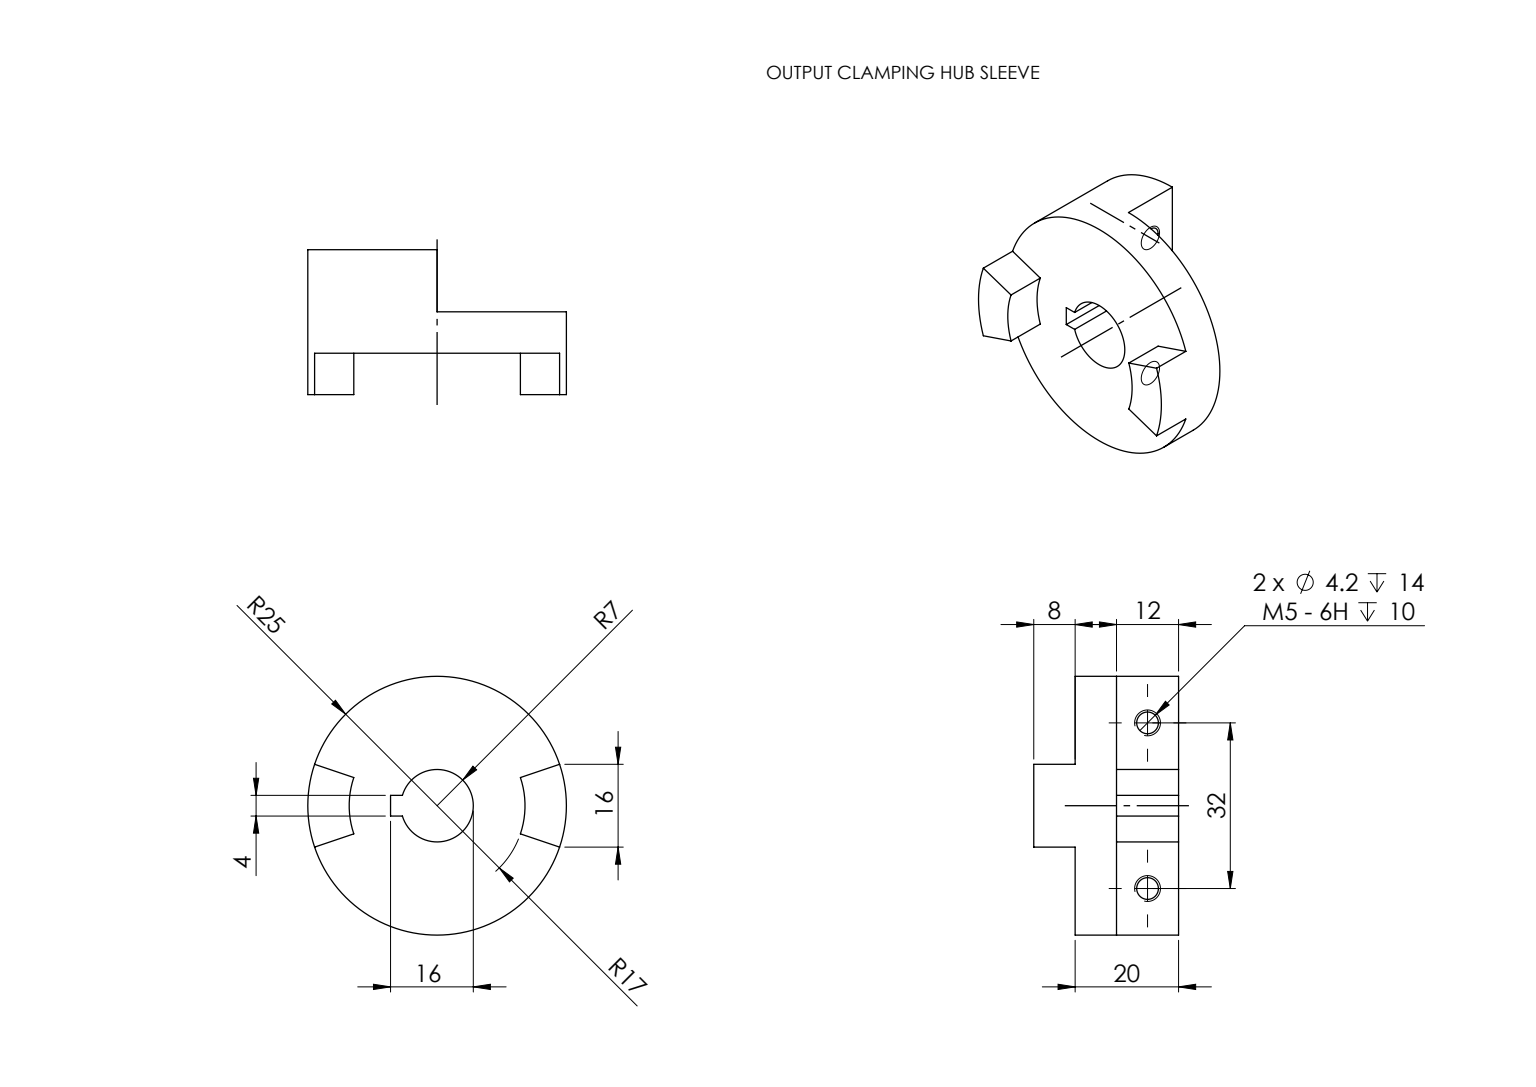
ISO-10303-21;
HEADER;
FILE_DESCRIPTION (('STEP AP214'),
    '1' );
FILE_NAME ('Output Clamping Hub Sleeve.step',
    '2026-10-08T14:09:18',
    ( '' ),
    ( '' ),
    'SwSTEP 2.0',
    'SolidWorks 2026',
    '' );
FILE_SCHEMA (( 'AUTOMOTIVE_DESIGN' ));
ENDSEC;

DATA;
#2=CARTESIAN_POINT ( 'NONE',  ( -6.517431832507181422E-14, 16.00000000000000000, -26.00000000000000355 ) ) ;
#4=CARTESIAN_POINT ( 'NONE',  ( 0.000000000000000000, 0.000000000000000000, -12.00000000000000000 ) ) ;
#5=AXIS2_PLACEMENT_3D ( 'NONE', #3716, #3077, #4925 ) ;
#9=VERTEX_POINT ( 'NONE', #2215 ) ;
#26=FACE_OUTER_BOUND ( 'NONE', #3587, .T. ) ;
#42=ORIENTED_EDGE ( 'NONE', *, *, #4705, .F. ) ;
#48=EDGE_LOOP ( 'NONE', ( #130, #2080, #1685, #2442 ) ) ;
#49=LINE ( 'NONE', #3799, #2903 ) ;
#54=VERTEX_POINT ( 'NONE', #3686 ) ;
#58=FACE_OUTER_BOUND ( 'NONE', #389, .T. ) ;
#82=ORIENTED_EDGE ( 'NONE', *, *, #1120, .T. ) ;
#83=AXIS2_PLACEMENT_3D ( 'NONE', #3595, #2177, #3698 ) ;
#84=ORIENTED_EDGE ( 'NONE', *, *, #4675, .T. ) ;
#85=SURFACE_STYLE_FILL_AREA ( #4292 ) ;
#95=ORIENTED_EDGE ( 'NONE', *, *, #1051, .F. ) ;
#97=VECTOR ( 'NONE', #3015, 1000.000000000000000 ) ;
#100=CIRCLE ( 'NONE', #2908, 6.999999999999999112 ) ;
#103=VECTOR ( 'NONE', #177, 1000.000000000000114 ) ;
#109=CIRCLE ( 'NONE', #436, 17.00000000000000000 ) ;
#112=CARTESIAN_POINT ( 'NONE',  ( 0.000000000000000000, 0.000000000000000000, -20.00000000000000000 ) ) ;
#116=CARTESIAN_POINT ( 'NONE',  ( -25.00000000000000000, 3.061616997868383043E-15, -4.000000000000000000 ) ) ;
#121=VERTEX_POINT ( 'NONE', #126 ) ;
#124=CARTESIAN_POINT ( 'NONE',  ( 16.10609822396473945, -5.439999999999995062, -4.000000000000000000 ) ) ;
#126=CARTESIAN_POINT ( 'NONE',  ( -16.10609822396473945, -5.439999999999995062, -12.00000000000000000 ) ) ;
#130=ORIENTED_EDGE ( 'NONE', *, *, #800, .F. ) ;
#135=DIRECTION ( 'NONE',  ( 0.5150380749100544886, 0.000000000000000000, -0.8571673007021121116 ) ) ;
#143=ORIENTED_EDGE ( 'NONE', *, *, #299, .T. ) ;
#144=DIRECTION ( 'NONE',  ( 1.000000000000000000, -0.000000000000000000, -0.000000000000000000 ) ) ;
#148=VERTEX_POINT ( 'NONE', #905 ) ;
#150=DIRECTION ( 'NONE',  ( -1.000000000000000000, -4.073394895316987600E-15, 0.000000000000000000 ) ) ;
#151=LINE ( 'NONE', #2483, #3855 ) ;
#161=DIRECTION ( 'NONE',  ( -1.000000000000000000, 0.000000000000000000, -0.000000000000000000 ) ) ;
#168=CARTESIAN_POINT ( 'NONE',  ( 23.68543856465402442, -8.000000000000003553, 14.30577747056276472 ) ) ;
#170=ORIENTED_EDGE ( 'NONE', *, *, #708, .F. ) ;
#171=CIRCLE ( 'NONE', #2417, 17.00000000000000000 ) ;
#174=EDGE_CURVE ( 'NONE', #4395, #54, #1471, .T. ) ;
#175=DIRECTION ( 'NONE',  ( 0.9474175425861609545, -0.3199999999999996181, 0.000000000000000000 ) ) ;
#177=DIRECTION ( 'NONE',  ( -0.9474175425861605104, 0.3200000000000010059, 0.000000000000000000 ) ) ;
#185=CARTESIAN_POINT ( 'NONE',  ( 16.10609822396473945, -5.439999999999995062, 14.30577747056276472 ) ) ;
#187=AXIS2_PLACEMENT_3D ( 'NONE', #4125, #819, #1824 ) ;
#189=ORIENTED_EDGE ( 'NONE', *, *, #3151, .T. ) ;
#194=DIRECTION ( 'NONE',  ( 0.000000000000000000, 0.000000000000000000, -1.000000000000000000 ) ) ;
#195=DIRECTION ( 'NONE',  ( -0.9474175425861605104, 0.3200000000000010059, 0.000000000000000000 ) ) ;
#196=EDGE_CURVE ( 'NONE', #2273, #1203, #931, .T. ) ;
#202=MECHANICAL_DESIGN_GEOMETRIC_PRESENTATION_REPRESENTATION('',(#2202),#282);
#210=DIRECTION ( 'NONE',  ( 0.000000000000000000, 0.000000000000000000, -1.000000000000000000 ) ) ;
#217=CARTESIAN_POINT ( 'NONE',  ( -13.99999999999993250, -16.00000000000000000, -26.00000000000000355 ) ) ;
#226=ORIENTED_EDGE ( 'NONE', *, *, #3828, .F. ) ;
#236=VECTOR ( 'NONE', #1592, 1000.000000000000000 ) ;
#238=DIRECTION ( 'NONE',  ( 1.000000000000000000, -0.000000000000000000, -0.000000000000000000 ) ) ;
#242=AXIS2_PLACEMENT_3D ( 'NONE', #3899, #3088, #3132 ) ;
#245=CIRCLE ( 'NONE', #405, 25.00000000000000000 ) ;
#251=DIRECTION ( 'NONE',  ( 1.000000000000000000, 0.000000000000000000, -0.000000000000000000 ) ) ;
#253=CIRCLE ( 'NONE', #5, 2.099999999999997868 ) ;
#254=AXIS2_PLACEMENT_3D ( 'NONE', #4822, #3198, #2921 ) ;
#261=AXIS2_PLACEMENT_3D ( 'NONE', #1866, #4851, #4564 ) ;
#265=( NAMED_UNIT ( * ) PLANE_ANGLE_UNIT ( ) SI_UNIT ( $, .RADIAN. ) );
#267=DIRECTION ( 'NONE',  ( 0.000000000000000000, -1.000000000000000000, 0.000000000000000000 ) ) ;
#269=LINE ( 'NONE', #4370, #3848 ) ;
#277=CARTESIAN_POINT ( 'NONE',  ( 0.000000000000000000, 0.000000000000000000, -12.00000000000000000 ) ) ;
#279=AXIS2_PLACEMENT_3D ( 'NONE', #4796, #2900, #4321 ) ;
#282=( GEOMETRIC_REPRESENTATION_CONTEXT ( 3 ) GLOBAL_UNCERTAINTY_ASSIGNED_CONTEXT ( ( #2248 ) ) GLOBAL_UNIT_ASSIGNED_CONTEXT ( ( #695, #1844, #4603 ) ) REPRESENTATION_CONTEXT ( 'NONE', 'WORKASPACE' ) );
#286=ORIENTED_EDGE ( 'NONE', *, *, #2509, .T. ) ;
#288=EDGE_CURVE ( 'NONE', #1390, #3410, #3646, .T. ) ;
#299=EDGE_CURVE ( 'NONE', #4175, #811, #2955, .T. ) ;
#319=PLANE ( 'NONE',  #4799 ) ;
#323=EDGE_CURVE ( 'NONE', #1722, #1339, #2532, .T. ) ;
#324=EDGE_LOOP ( 'NONE', ( #3270, #945 ) ) ;
#326=CARTESIAN_POINT ( 'NONE',  ( 0.000000000000000000, 25.00000000000000000, -20.00000000000000000 ) ) ;
#336=CARTESIAN_POINT ( 'NONE',  ( -7.332110811570578784E-14, -6.999999999999999112, -32.00000000000000000 ) ) ;
#344=FACE_OUTER_BOUND ( 'NONE', #964, .T. ) ;
#351=DIRECTION ( 'NONE',  ( 0.9474175425861605104, 0.3200000000000010059, 0.000000000000000000 ) ) ;
#353=SURFACE_STYLE_FILL_AREA ( #4217 ) ;
#357=DIRECTION ( 'NONE',  ( 0.9474175425861609545, 0.3199999999999996181, -0.000000000000000000 ) ) ;
#359=DIRECTION ( 'NONE',  ( -0.000000000000000000, -0.000000000000000000, 1.000000000000000000 ) ) ;
#367=ORIENTED_EDGE ( 'NONE', *, *, #4173, .F. ) ;
#378=DIRECTION ( 'NONE',  ( 1.000000000000000000, -0.000000000000000000, -0.000000000000000000 ) ) ;
#388=ORIENTED_EDGE ( 'NONE', *, *, #3153, .T. ) ;
#389=EDGE_LOOP ( 'NONE', ( #2947, #665, #449, #3173, #4854, #2496, #2657, #940, #4548 ) ) ;
#396=CIRCLE ( 'NONE', #2236, 25.00000000000000000 ) ;
#399=CIRCLE ( 'NONE', #3208, 2.099999999999997868 ) ;
#405=AXIS2_PLACEMENT_3D ( 'NONE', #4519, #1873, #1469 ) ;
#407=VECTOR ( 'NONE', #816, 1000.000000000000000 ) ;
#411=CARTESIAN_POINT ( 'NONE',  ( 0.000000000000000000, 0.000000000000000000, -20.00000000000000000 ) ) ;
#413=AXIS2_PLACEMENT_3D ( 'NONE', #411, #1607, #4207 ) ;
#415=ORIENTED_EDGE ( 'NONE', *, *, #196, .T. ) ;
#419=DIRECTION ( 'NONE',  ( -0.000000000000000000, -0.000000000000000000, -1.000000000000000000 ) ) ;
#425=MANIFOLD_SOLID_BREP ( 'M5 Tapped Hole1', #4581 ) ;
#431=DIRECTION ( 'NONE',  ( 0.000000000000000000, 0.000000000000000000, -1.000000000000000000 ) ) ;
#436=AXIS2_PLACEMENT_3D ( 'NONE', #2401, #1271, #4371 ) ;
#449=ORIENTED_EDGE ( 'NONE', *, *, #2315, .T. ) ;
#460=ORIENTED_EDGE ( 'NONE', *, *, #523, .T. ) ;
#462=EDGE_CURVE ( 'NONE', #3903, #3640, #245, .T. ) ;
#469=ADVANCED_BREP_SHAPE_REPRESENTATION ( '', ( #425, #1918 ), #4450 ) ;
#474=( NAMED_UNIT ( * ) SI_UNIT ( $, .STERADIAN. ) SOLID_ANGLE_UNIT ( ) );
#476=DIRECTION ( 'NONE',  ( 0.000000000000000000, 0.000000000000000000, -1.000000000000000000 ) ) ;
#479=VERTEX_POINT ( 'NONE', #1438 ) ;
#483=ADVANCED_FACE ( 'NONE', ( #2985 ), #1043, .F. ) ;
#491=ORIENTED_EDGE ( 'NONE', *, *, #4912, .F. ) ;
#495=LINE ( 'NONE', #1938, #2572 ) ;
#496=CYLINDRICAL_SURFACE ( 'NONE', #2581, 6.999999999999999112 ) ;
#498=AXIS2_PLACEMENT_3D ( 'NONE', #873, #431, #3187 ) ;
#502=DIRECTION ( 'NONE',  ( -0.000000000000000000, -0.000000000000000000, 1.000000000000000000 ) ) ;
#507=DIRECTION ( 'NONE',  ( -1.000000000000000000, 0.000000000000000000, 0.000000000000000000 ) ) ;
#509=ORIENTED_EDGE ( 'NONE', *, *, #4882, .F. ) ;
#511=CIRCLE ( 'NONE', #1053, 6.999999999999999112 ) ;
#518=CIRCLE ( 'NONE', #1149, 17.00000000000000000 ) ;
#520=DIRECTION ( 'NONE',  ( 0.000000000000000000, 0.000000000000000000, -1.000000000000000000 ) ) ;
#523=EDGE_CURVE ( 'NONE', #852, #654, #2199, .T. ) ;
#524=ORIENTED_EDGE ( 'NONE', *, *, #2305, .F. ) ;
#530=ORIENTED_EDGE ( 'NONE', *, *, #1162, .F. ) ;
#536=VERTEX_POINT ( 'NONE', #1955 ) ;
#537=VERTEX_POINT ( 'NONE', #3576 ) ;
#544=( NAMED_UNIT ( * ) PLANE_ANGLE_UNIT ( ) SI_UNIT ( $, .RADIAN. ) );
#545=PLANE ( 'NONE',  #2901 ) ;
#546=DIRECTION ( 'NONE',  ( -0.000000000000000000, -0.000000000000000000, 1.000000000000000000 ) ) ;
#551=CARTESIAN_POINT ( 'NONE',  ( -7.332110811570578784E-14, -6.999999999999999112, -32.00000000000000000 ) ) ;
#554=DIRECTION ( 'NONE',  ( -0.9474175425861605104, -0.3200000000000010059, 0.000000000000000000 ) ) ;
#561=DIRECTION ( 'NONE',  ( 1.000000000000000000, -1.892318758829013864E-15, 0.000000000000000000 ) ) ;
#565=CARTESIAN_POINT ( 'NONE',  ( 23.68543856465402442, -8.000000000000003553, -4.000000000000000000 ) ) ;
#567=ORIENTED_EDGE ( 'NONE', *, *, #4261, .F. ) ;
#573=CARTESIAN_POINT ( 'NONE',  ( -17.00000000000000000, 0.000000000000000000, 14.30577747056276472 ) ) ;
#576=VECTOR ( 'NONE', #357, 1000.000000000000114 ) ;
#579=AXIS2_PLACEMENT_3D ( 'NONE', #2046, #3223, #4745 ) ;
#584=EDGE_LOOP ( 'NONE', ( #3424, #607, #226, #4068, #1963 ) ) ;
#589=ORIENTED_EDGE ( 'NONE', *, *, #3682, .F. ) ;
#593=CARTESIAN_POINT ( 'NONE',  ( -9.000000000000001776, 2.000000000000000000, -20.00000000000000000 ) ) ;
#597=VERTEX_POINT ( 'NONE', #124 ) ;
#600=PRODUCT_CONTEXT ( 'NONE', #768, 'mechanical' ) ;
#607=ORIENTED_EDGE ( 'NONE', *, *, #1884, .F. ) ;
#611=DIRECTION ( 'NONE',  ( -1.000000000000000000, 0.000000000000000000, 0.000000000000000000 ) ) ;
#624=LINE ( 'NONE', #3677, #576 ) ;
#626=LINE ( 'NONE', #4130, #2829 ) ;
#627=ORIENTED_EDGE ( 'NONE', *, *, #2610, .F. ) ;
#630=( LENGTH_UNIT ( ) NAMED_UNIT ( * ) SI_UNIT ( .MILLI., .METRE. ) );
#631=CIRCLE ( 'NONE', #3433, 25.00000000000000000 ) ;
#633=CARTESIAN_POINT ( 'NONE',  ( -6.517431832507181422E-14, 16.00000000000000000, -28.10000000000000142 ) ) ;
#637=DIRECTION ( 'NONE',  ( 0.000000000000000000, 0.000000000000000000, -1.000000000000000000 ) ) ;
#642=CARTESIAN_POINT ( 'NONE',  ( -13.99999999999993250, -16.00000000000000000, -26.00000000000000355 ) ) ;
#653=CIRCLE ( 'NONE', #3857, 2.099999999999997868 ) ;
#654=VERTEX_POINT ( 'NONE', #4651 ) ;
#658=PLANE ( 'NONE',  #2178 ) ;
#659=AXIS2_PLACEMENT_3D ( 'NONE', #1459, #3001, #4158 ) ;
#665=ORIENTED_EDGE ( 'NONE', *, *, #2003, .T. ) ;
#674=COLOUR_RGB ( '', 0.09019608, 0.27058824, 0.51372549) ;
#689=CARTESIAN_POINT ( 'NONE',  ( 16.10609822396473589, 5.440000000000003055, -4.000000000000000000 ) ) ;
#694=DIRECTION ( 'NONE',  ( 0.000000000000000000, 0.000000000000000000, -1.000000000000000000 ) ) ;
#695=( LENGTH_UNIT ( ) NAMED_UNIT ( * ) SI_UNIT ( .MILLI., .METRE. ) );
#701=ORIENTED_EDGE ( 'NONE', *, *, #4533, .T. ) ;
#707=ORIENTED_EDGE ( 'NONE', *, *, #765, .F. ) ;
#708=EDGE_CURVE ( 'NONE', #2396, #2782, #2504, .T. ) ;
#713=AXIS2_PLACEMENT_3D ( 'NONE', #1995, #4324, #507 ) ;
#720=VECTOR ( 'NONE', #1698, 1000.000000000000000 ) ;
#724=CARTESIAN_POINT ( 'NONE',  ( 6.497531322021036645E-14, -16.00000000000000000, -23.90000000000000568 ) ) ;
#731=DIRECTION ( 'NONE',  ( -0.000000000000000000, -0.000000000000000000, 1.000000000000000000 ) ) ;
#757=CARTESIAN_POINT ( 'NONE',  ( 0.000000000000000000, -1.999999999999999112, -20.00000000000000000 ) ) ;
#758=CYLINDRICAL_SURFACE ( 'NONE', #3930, 2.099999999999997868 ) ;
#765=EDGE_CURVE ( 'NONE', #148, #1558, #1764, .T. ) ;
#768=APPLICATION_CONTEXT ( 'automotive_design' ) ;
#782=ORIENTED_EDGE ( 'NONE', *, *, #2643, .T. ) ;
#790=UNCERTAINTY_MEASURE_WITH_UNIT (LENGTH_MEASURE( 1.000000000000000082E-05 ), #921, 'distance_accuracy_value', 'NONE');
#800=EDGE_CURVE ( 'NONE', #3536, #4716, #4237, .T. ) ;
#806=DIRECTION ( 'NONE',  ( -0.000000000000000000, -0.000000000000000000, 1.000000000000000000 ) ) ;
#809=VECTOR ( 'NONE', #2774, 1000.000000000000000 ) ;
#811=VERTEX_POINT ( 'NONE', #4516 ) ;
#815=CIRCLE ( 'NONE', #1850, 2.099999999999997868 ) ;
#816=DIRECTION ( 'NONE',  ( 0.5150380749100544886, 1.049727191138618449E-16, 0.8571673007021121116 ) ) ;
#819=DIRECTION ( 'NONE',  ( 0.000000000000000000, 0.000000000000000000, 1.000000000000000000 ) ) ;
#822=VECTOR ( 'NONE', #3608, 1000.000000000000114 ) ;
#850=LINE ( 'NONE', #4216, #4959 ) ;
#852=VERTEX_POINT ( 'NONE', #2573 ) ;
#865=VERTEX_POINT ( 'NONE', #3009 ) ;
#867=DIRECTION ( 'NONE',  ( 1.000000000000000000, -0.000000000000000000, -0.000000000000000000 ) ) ;
#873=CARTESIAN_POINT ( 'NONE',  ( 0.000000000000000000, 0.000000000000000000, -20.00000000000000000 ) ) ;
#891=CARTESIAN_POINT ( 'NONE',  ( 0.000000000000000000, 0.000000000000000000, -12.00000000000000000 ) ) ;
#897=DIRECTION ( 'NONE',  ( -0.000000000000000000, -0.000000000000000000, -1.000000000000000000 ) ) ;
#901=VECTOR ( 'NONE', #135, 1000.000000000000000 ) ;
#903=ORIENTED_EDGE ( 'NONE', *, *, #1204, .T. ) ;
#905=CARTESIAN_POINT ( 'NONE',  ( 23.68543856465402442, -8.000000000000003553, -4.000000000000000000 ) ) ;
#910=LINE ( 'NONE', #1678, #1139 ) ;
#911=EDGE_LOOP ( 'NONE', ( #4750, #2184, #415, #388 ) ) ;
#921=( LENGTH_UNIT ( ) NAMED_UNIT ( * ) SI_UNIT ( .MILLI., .METRE. ) );
#927=CARTESIAN_POINT ( 'NONE',  ( -9.000000000000003553, -1.999999999999999112, -12.00000000000000000 ) ) ;
#931=LINE ( 'NONE', #2457, #3169 ) ;
#937=LINE ( 'NONE', #3914, #2427 ) ;
#940=ORIENTED_EDGE ( 'NONE', *, *, #4943, .T. ) ;
#945=ORIENTED_EDGE ( 'NONE', *, *, #2751, .F. ) ;
#948=ORIENTED_EDGE ( 'NONE', *, *, #4220, .T. ) ;
#951=CARTESIAN_POINT ( 'NONE',  ( -6.537332342993324937E-14, 16.00000000000000000, -26.00000000000000355 ) ) ;
#962=DIRECTION ( 'NONE',  ( 0.000000000000000000, 0.000000000000000000, -1.000000000000000000 ) ) ;
#964=EDGE_LOOP ( 'NONE', ( #3898, #1479, #2019, #627, #4843, #4193 ) ) ;
#968=CIRCLE ( 'NONE', #4077, 25.00000000000000000 ) ;
#969=ORIENTED_EDGE ( 'NONE', *, *, #1204, .F. ) ;
#974=CARTESIAN_POINT ( 'NONE',  ( 0.000000000000000000, 0.000000000000000000, -12.00000000000000000 ) ) ;
#977=ORIENTED_EDGE ( 'NONE', *, *, #4608, .F. ) ;
#984=LINE ( 'NONE', #4405, #3775 ) ;
#991=VERTEX_POINT ( 'NONE', #116 ) ;
#1000=CARTESIAN_POINT ( 'NONE',  ( 16.10609822396473589, 5.440000000000003055, 14.30577747056276472 ) ) ;
#1007=CARTESIAN_POINT ( 'NONE',  ( -6.537332342993324937E-14, 16.00000000000000000, -26.00000000000000355 ) ) ;
#1016=PRODUCT ( 'Output Clamping Hub Sleeve', 'Output Clamping Hub Sleeve', '', ( #600 ) ) ;
#1017=CYLINDRICAL_SURFACE ( 'NONE', #1512, 17.00000000000000000 ) ;
#1021=MECHANICAL_DESIGN_GEOMETRIC_PRESENTATION_REPRESENTATION('',(#3423),#4138);
#1027=EDGE_CURVE ( 'NONE', #3993, #1343, #968, .T. ) ;
#1029=PLANE ( 'NONE',  #4821 ) ;
#1031=VERTEX_POINT ( 'NONE', #4319 ) ;
#1035=DIRECTION ( 'NONE',  ( 1.000000000000000000, -0.000000000000000000, -0.000000000000000000 ) ) ;
#1038=EDGE_LOOP ( 'NONE', ( #524, #589, #4148, #2680, #1210, #4780, #1790, #3348, #2804, #82 ) ) ;
#1041=DIRECTION ( 'NONE',  ( -0.000000000000000000, -0.000000000000000000, 1.000000000000000000 ) ) ;
#1043=CONICAL_SURFACE ( 'NONE', #1362, 2.099999999999997868, 1.029744258676654090 ) ;
#1051=EDGE_CURVE ( 'NONE', #1467, #479, #3496, .T. ) ;
#1053=AXIS2_PLACEMENT_3D ( 'NONE', #974, #3260, #3214 ) ;
#1058=AXIS2_PLACEMENT_3D ( 'NONE', #3400, #2679, #251 ) ;
#1063=CARTESIAN_POINT ( 'NONE',  ( -16.10609822396473589, 5.440000000000003055, -4.000000000000000000 ) ) ;
#1079=CARTESIAN_POINT ( 'NONE',  ( 0.000000000000000000, 25.00000000000000000, -32.00000000000000000 ) ) ;
#1082=FACE_OUTER_BOUND ( 'NONE', #3709, .T. ) ;
#1083=EDGE_LOOP ( 'NONE', ( #286, #4197, #170, #2268 ) ) ;
#1087=FACE_OUTER_BOUND ( 'NONE', #1306, .T. ) ;
#1090=ORIENTED_EDGE ( 'NONE', *, *, #3059, .T. ) ;
#1115=DIRECTION ( 'NONE',  ( 1.000000000000000000, 0.000000000000000000, 0.000000000000000000 ) ) ;
#1118=AXIS2_PLACEMENT_3D ( 'NONE', #3796, #3850, #2357 ) ;
#1120=EDGE_CURVE ( 'NONE', #1203, #991, #1604, .T. ) ;
#1122=DIRECTION ( 'NONE',  ( -0.000000000000000000, -0.000000000000000000, 1.000000000000000000 ) ) ;
#1139=VECTOR ( 'NONE', #2847, 1000.000000000000000 ) ;
#1144=AXIS2_PLACEMENT_3D ( 'NONE', #891, #2352, #3950 ) ;
#1146=CARTESIAN_POINT ( 'NONE',  ( 0.000000000000000000, 0.000000000000000000, 0.000000000000000000 ) ) ;
#1148=FACE_OUTER_BOUND ( 'NONE', #3721, .T. ) ;
#1149=AXIS2_PLACEMENT_3D ( 'NONE', #2228, #1470, #1993 ) ;
#1151=CYLINDRICAL_SURFACE ( 'NONE', #3829, 25.00000000000000000 ) ;
#1152=FILL_AREA_STYLE_COLOUR ( '', #674 ) ;
#1162=EDGE_CURVE ( 'NONE', #4131, #3536, #1946, .T. ) ;
#1170=EDGE_LOOP ( 'NONE', ( #1550, #3395, #4871, #3982 ) ) ;
#1171=CARTESIAN_POINT ( 'NONE',  ( 0.000000000000000000, 0.000000000000000000, -4.000000000000000000 ) ) ;
#1173=PLANE ( 'NONE',  #187 ) ;
#1178=ADVANCED_FACE ( 'NONE', ( #2145 ), #4808, .F. ) ;
#1182=EDGE_CURVE ( 'NONE', #4937, #2834, #3660, .T. ) ;
#1188=COLOUR_RGB ( '', 0.09019608, 0.27058824, 0.51372549) ;
#1203=VERTEX_POINT ( 'NONE', #4060 ) ;
#1204=EDGE_CURVE ( 'NONE', #1722, #1390, #2521, .T. ) ;
#1210=ORIENTED_EDGE ( 'NONE', *, *, #4882, .T. ) ;
#1215=DIRECTION ( 'NONE',  ( -0.000000000000000000, -0.000000000000000000, 1.000000000000000000 ) ) ;
#1223=FACE_OUTER_BOUND ( 'NONE', #4578, .T. ) ;
#1227=AXIS2_PLACEMENT_3D ( 'NONE', #2025, #867, #476 ) ;
#1228=FACE_OUTER_BOUND ( 'NONE', #3061, .T. ) ;
#1244=LINE ( 'NONE', #2091, #822 ) ;
#1261=ORIENTED_EDGE ( 'NONE', *, *, #3181, .T. ) ;
#1264=DIRECTION ( 'NONE',  ( 4.073394895316987600E-15, -1.000000000000000000, 0.000000000000000000 ) ) ;
#1266=EDGE_LOOP ( 'NONE', ( #3202, #3863, #2347, #3636 ) ) ;
#1271=DIRECTION ( 'NONE',  ( 0.000000000000000000, 0.000000000000000000, 1.000000000000000000 ) ) ;
#1284=AXIS2_PLACEMENT_3D ( 'NONE', #4119, #4902, #2527 ) ;
#1285=ORIENTED_EDGE ( 'NONE', *, *, #4911, .F. ) ;
#1289=FACE_OUTER_BOUND ( 'NONE', #4132, .T. ) ;
#1292=ORIENTED_EDGE ( 'NONE', *, *, #2610, .T. ) ;
#1293=CARTESIAN_POINT ( 'NONE',  ( -14.00000000000006395, 16.00000000000000000, -26.00000000000000355 ) ) ;
#1298=ORIENTED_EDGE ( 'NONE', *, *, #2437, .T. ) ;
#1305=CIRCLE ( 'NONE', #1144, 25.00000000000000000 ) ;
#1306=EDGE_LOOP ( 'NONE', ( #4774, #1285, #3515, #1292 ) ) ;
#1316=EDGE_CURVE ( 'NONE', #2020, #1912, #4082, .T. ) ;
#1319=VERTEX_POINT ( 'NONE', #3970 ) ;
#1329=ADVANCED_FACE ( 'NONE', ( #2541 ), #545, .T. ) ;
#1336=FACE_OUTER_BOUND ( 'NONE', #4607, .T. ) ;
#1339=VERTEX_POINT ( 'NONE', #1063 ) ;
#1341=CARTESIAN_POINT ( 'NONE',  ( -13.99999999999993250, -16.00000000000000000, -26.00000000000000355 ) ) ;
#1343=VERTEX_POINT ( 'NONE', #4509 ) ;
#1355=ORIENTED_EDGE ( 'NONE', *, *, #3411, .T. ) ;
#1362=AXIS2_PLACEMENT_3D ( 'NONE', #1897, #3377, #2606 ) ;
#1364=CARTESIAN_POINT ( 'NONE',  ( 25.00000000000000000, 0.000000000000000000, -20.00000000000000000 ) ) ;
#1368=CIRCLE ( 'NONE', #2824, 6.999999999999999112 ) ;
#1376=AXIS2_PLACEMENT_3D ( 'NONE', #3753, #4202, #3409 ) ;
#1377=APPLICATION_CONTEXT ( 'automotive_design' ) ;
#1387=DIRECTION ( 'NONE',  ( 0.000000000000000000, 0.000000000000000000, -1.000000000000000000 ) ) ;
#1389=DIRECTION ( 'NONE',  ( 1.000000000000000000, -0.000000000000000000, -0.000000000000000000 ) ) ;
#1390=VERTEX_POINT ( 'NONE', #2638 ) ;
#1412=CYLINDRICAL_SURFACE ( 'NONE', #261, 6.999999999999999112 ) ;
#1421=ADVANCED_FACE ( 'NONE', ( #3392 ), #658, .F. ) ;
#1433=FACE_OUTER_BOUND ( 'NONE', #1585, .T. ) ;
#1436=ORIENTED_EDGE ( 'NONE', *, *, #1447, .F. ) ;
#1438=CARTESIAN_POINT ( 'NONE',  ( 6.497531322021036645E-14, -16.00000000000000000, -28.10000000000000142 ) ) ;
#1441=VECTOR ( 'NONE', #3616, 1000.000000000000000 ) ;
#1447=EDGE_CURVE ( 'NONE', #2396, #654, #4893, .T. ) ;
#1451=CARTESIAN_POINT ( 'NONE',  ( 2.444036937190193033E-14, 6.999999999999999112, -20.00000000000000000 ) ) ;
#1455=EDGE_LOOP ( 'NONE', ( #42, #2415, #3096, #2460 ) ) ;
#1457=AXIS2_PLACEMENT_3D ( 'NONE', #1971, #2989, #3498 ) ;
#1459=CARTESIAN_POINT ( 'NONE',  ( -4.336808689942023652E-16, 2.000000000000002220, -20.00000000000000000 ) ) ;
#1467=VERTEX_POINT ( 'NONE', #3787 ) ;
#1469=DIRECTION ( 'NONE',  ( -1.000000000000000000, 0.000000000000000000, 0.000000000000000000 ) ) ;
#1470=DIRECTION ( 'NONE',  ( 0.000000000000000000, 0.000000000000000000, 1.000000000000000000 ) ) ;
#1471=CIRCLE ( 'NONE', #4031, 6.999999999999999112 ) ;
#1473=LINE ( 'NONE', #326, #97 ) ;
#1479=ORIENTED_EDGE ( 'NONE', *, *, #4639, .T. ) ;
#1499=ORIENTED_EDGE ( 'NONE', *, *, #299, .F. ) ;
#1512=AXIS2_PLACEMENT_3D ( 'NONE', #2201, #637, #3326 ) ;
#1522=DIRECTION ( 'NONE',  ( -1.000000000000000000, -3.784637517658031179E-16, -0.000000000000000000 ) ) ;
#1531=DIRECTION ( 'NONE',  ( 0.000000000000000000, 0.000000000000000000, -1.000000000000000000 ) ) ;
#1550=ORIENTED_EDGE ( 'NONE', *, *, #4235, .T. ) ;
#1555=PLANE ( 'NONE',  #2113 ) ;
#1557=LINE ( 'NONE', #4611, #4253 ) ;
#1558=VERTEX_POINT ( 'NONE', #4592 ) ;
#1562=DIRECTION ( 'NONE',  ( -1.000000000000000000, 0.000000000000000000, -0.000000000000000000 ) ) ;
#1567=ORIENTED_EDGE ( 'NONE', *, *, #1945, .F. ) ;
#1578=DIRECTION ( 'NONE',  ( 1.000000000000000000, 2.168404344971009361E-16, 0.000000000000000000 ) ) ;
#1583=CARTESIAN_POINT ( 'NONE',  ( -7.332110811570578784E-14, -6.999999999999999112, -20.00000000000000000 ) ) ;
#1585=EDGE_LOOP ( 'NONE', ( #1499, #1942, #2195, #3333 ) ) ;
#1592=DIRECTION ( 'NONE',  ( 1.000000000000000000, -0.000000000000000000, -0.000000000000000000 ) ) ;
#1599=CARTESIAN_POINT ( 'NONE',  ( -4.336808689942023652E-16, 2.000000000000002220, -12.00000000000000000 ) ) ;
#1604=CIRCLE ( 'NONE', #3762, 25.00000000000000000 ) ;
#1607=DIRECTION ( 'NONE',  ( -0.000000000000000000, -0.000000000000000000, 1.000000000000000000 ) ) ;
#1614=SURFACE_SIDE_STYLE ('',( #85 ) ) ;
#1630=DIRECTION ( 'NONE',  ( 4.073394895316987600E-15, -1.000000000000000000, 0.000000000000000000 ) ) ;
#1645=EDGE_CURVE ( 'NONE', #1339, #3410, #2044, .T. ) ;
#1647=DIRECTION ( 'NONE',  ( -0.000000000000000000, -0.000000000000000000, -1.000000000000000000 ) ) ;
#1653=LINE ( 'NONE', #4734, #103 ) ;
#1660=ORIENTED_EDGE ( 'NONE', *, *, #1996, .T. ) ;
#1669=EDGE_CURVE ( 'NONE', #597, #1031, #1681, .T. ) ;
#1672=EDGE_LOOP ( 'NONE', ( #3004, #3131, #3882, #3418 ) ) ;
#1678=CARTESIAN_POINT ( 'NONE',  ( -23.68543856465402442, -8.000000000000003553, 14.30577747056276472 ) ) ;
#1681=LINE ( 'NONE', #185, #1934 ) ;
#1685=ORIENTED_EDGE ( 'NONE', *, *, #2751, .T. ) ;
#1690=DIRECTION ( 'NONE',  ( -1.000000000000000000, 0.000000000000000000, 0.000000000000000000 ) ) ;
#1691=VECTOR ( 'NONE', #731, 1000.000000000000000 ) ;
#1697=DIRECTION ( 'NONE',  ( 1.357798298438996130E-15, -1.000000000000000000, 0.000000000000000000 ) ) ;
#1698=DIRECTION ( 'NONE',  ( 4.073394895316987600E-15, -1.000000000000000000, 0.000000000000000000 ) ) ;
#1715=VECTOR ( 'NONE', #2134, 1000.000000000000114 ) ;
#1722=VERTEX_POINT ( 'NONE', #4383 ) ;
#1729=DIRECTION ( 'NONE',  ( -4.336808689942018722E-16, -1.000000000000000000, 0.000000000000000000 ) ) ;
#1735=FACE_OUTER_BOUND ( 'NONE', #1170, .T. ) ;
#1757=FACE_OUTER_BOUND ( 'NONE', #3032, .T. ) ;
#1760=EDGE_LOOP ( 'NONE', ( #189, #4344, #367, #1298 ) ) ;
#1764=LINE ( 'NONE', #168, #1840 ) ;
#1774=PRODUCT_DEFINITION_SHAPE ( 'NONE', 'NONE',  #2896 ) ;
#1775=ORIENTED_EDGE ( 'NONE', *, *, #323, .T. ) ;
#1781=DIRECTION ( 'NONE',  ( 1.000000000000000000, -0.000000000000000000, -0.000000000000000000 ) ) ;
#1783=CIRCLE ( 'NONE', #2761, 25.00000000000000000 ) ;
#1786=CARTESIAN_POINT ( 'NONE',  ( 0.000000000000000000, 0.000000000000000000, -12.00000000000000000 ) ) ;
#1790=ORIENTED_EDGE ( 'NONE', *, *, #765, .T. ) ;
#1794=DIRECTION ( 'NONE',  ( 1.000000000000000000, -0.000000000000000000, -0.000000000000000000 ) ) ;
#1803=LINE ( 'NONE', #3332, #2185 ) ;
#1810=( NAMED_UNIT ( * ) SI_UNIT ( $, .STERADIAN. ) SOLID_ANGLE_UNIT ( ) );
#1814=CARTESIAN_POINT ( 'NONE',  ( 2.444036937190193033E-14, 6.999999999999999112, -32.00000000000000000 ) ) ;
#1824=DIRECTION ( 'NONE',  ( 1.000000000000000000, 0.000000000000000000, -0.000000000000000000 ) ) ;
#1836=DIRECTION ( 'NONE',  ( 0.000000000000000000, 0.000000000000000000, -1.000000000000000000 ) ) ;
#1840=VECTOR ( 'NONE', #4831, 1000.000000000000000 ) ;
#1844=( NAMED_UNIT ( * ) PLANE_ANGLE_UNIT ( ) SI_UNIT ( $, .RADIAN. ) );
#1850=AXIS2_PLACEMENT_3D ( 'NONE', #1007, #3965, #2141 ) ;
#1852=PLANE ( 'NONE',  #2825 ) ;
#1853=ADVANCED_FACE ( 'NONE', ( #4885, #2557 ), #1852, .F. ) ;
#1857=VECTOR ( 'NONE', #1522, 1000.000000000000000 ) ;
#1866=CARTESIAN_POINT ( 'NONE',  ( 0.000000000000000000, 0.000000000000000000, -20.00000000000000000 ) ) ;
#1872=CARTESIAN_POINT ( 'NONE',  ( -6.708203932499367639, 2.000000000000001332, -32.00000000000000000 ) ) ;
#1873=DIRECTION ( 'NONE',  ( 0.000000000000000000, 0.000000000000000000, -1.000000000000000000 ) ) ;
#1879=DIRECTION ( 'NONE',  ( -1.000000000000000000, 0.000000000000000000, 0.000000000000000000 ) ) ;
#1884=EDGE_CURVE ( 'NONE', #4842, #3993, #624, .T. ) ;
#1897=CARTESIAN_POINT ( 'NONE',  ( -13.99999999999993250, -16.00000000000000000, -26.00000000000000355 ) ) ;
#1909=CARTESIAN_POINT ( 'NONE',  ( 0.000000000000000000, 0.000000000000000000, -12.00000000000000000 ) ) ;
#1910=EDGE_CURVE ( 'NONE', #3903, #4259, #1473, .T. ) ;
#1912=VERTEX_POINT ( 'NONE', #4524 ) ;
#1914=ORIENTED_EDGE ( 'NONE', *, *, #4729, .T. ) ;
#1918=AXIS2_PLACEMENT_3D ( 'NONE', #1146, #2700, #1115 ) ;
#1920=DIRECTION ( 'NONE',  ( -0.000000000000000000, -0.000000000000000000, 1.000000000000000000 ) ) ;
#1929=CARTESIAN_POINT ( 'NONE',  ( -16.10609822396473589, 5.440000000000003055, -12.00000000000000000 ) ) ;
#1934=VECTOR ( 'NONE', #520, 1000.000000000000000 ) ;
#1938=CARTESIAN_POINT ( 'NONE',  ( -1.387778780781444295E-15, 4.108768631691174362E-15, -12.00000000000000000 ) ) ;
#1942=ORIENTED_EDGE ( 'NONE', *, *, #3742, .T. ) ;
#1945=EDGE_CURVE ( 'NONE', #3993, #4372, #49, .T. ) ;
#1946=LINE ( 'NONE', #4239, #407 ) ;
#1955=CARTESIAN_POINT ( 'NONE',  ( -6.537332342993324937E-14, 16.00000000000000000, -28.10000000000000142 ) ) ;
#1960=DIRECTION ( 'NONE',  ( 0.000000000000000000, 0.000000000000000000, -1.000000000000000000 ) ) ;
#1963=ORIENTED_EDGE ( 'NONE', *, *, #4785, .F. ) ;
#1969=CARTESIAN_POINT ( 'NONE',  ( 6.517431832507181422E-14, -16.00000000000000000, -28.10000000000000142 ) ) ;
#1971=CARTESIAN_POINT ( 'NONE',  ( 0.000000000000000000, 0.000000000000000000, -32.00000000000000000 ) ) ;
#1993=DIRECTION ( 'NONE',  ( 1.000000000000000000, 0.000000000000000000, 0.000000000000000000 ) ) ;
#1994=ORIENTED_EDGE ( 'NONE', *, *, #4912, .T. ) ;
#1995=CARTESIAN_POINT ( 'NONE',  ( 0.000000000000000000, 0.000000000000000000, 14.30577747056276472 ) ) ;
#1996=EDGE_CURVE ( 'NONE', #54, #4892, #511, .T. ) ;
#2003=EDGE_CURVE ( 'NONE', #1558, #1031, #1653, .T. ) ;
#2008=EDGE_LOOP ( 'NONE', ( #567, #948, #701 ) ) ;
#2010=EDGE_CURVE ( 'NONE', #536, #865, #653, .T. ) ;
#2011=VECTOR ( 'NONE', #1387, 1000.000000000000000 ) ;
#2012=ADVANCED_FACE ( 'NONE', ( #1148 ), #4426, .T. ) ;
#2019=ORIENTED_EDGE ( 'NONE', *, *, #174, .F. ) ;
#2020=VERTEX_POINT ( 'NONE', #3054 ) ;
#2025=CARTESIAN_POINT ( 'NONE',  ( 6.517431832507181422E-14, -16.00000000000000000, -26.00000000000000355 ) ) ;
#2027=ORIENTED_EDGE ( 'NONE', *, *, #523, .F. ) ;
#2034=ORIENTED_EDGE ( 'NONE', *, *, #3416, .F. ) ;
#2044=LINE ( 'NONE', #2486, #3939 ) ;
#2046=CARTESIAN_POINT ( 'NONE',  ( 23.68543856465402797, 7.999999999999996447, 14.30577747056276472 ) ) ;
#2067=DIRECTION ( 'NONE',  ( -4.336808689942018722E-16, -1.000000000000000000, 0.000000000000000000 ) ) ;
#2070=ORIENTED_EDGE ( 'NONE', *, *, #1910, .F. ) ;
#2071=CARTESIAN_POINT ( 'NONE',  ( 0.000000000000000000, 0.000000000000000000, -20.00000000000000000 ) ) ;
#2080=ORIENTED_EDGE ( 'NONE', *, *, #4705, .T. ) ;
#2081=CIRCLE ( 'NONE', #4149, 2.099999999999997868 ) ;
#2086=VECTOR ( 'NONE', #1041, 1000.000000000000000 ) ;
#2091=CARTESIAN_POINT ( 'NONE',  ( -7.216449660063538023E-15, 2.136559688479409280E-14, -12.00000000000000000 ) ) ;
#2097=DIRECTION ( 'NONE',  ( 0.000000000000000000, 0.000000000000000000, -1.000000000000000000 ) ) ;
#2109=EDGE_LOOP ( 'NONE', ( #2650, #1660, #2686, #4663, #1090 ) ) ;
#2113=AXIS2_PLACEMENT_3D ( 'NONE', #4128, #3800, #4584 ) ;
#2114=CARTESIAN_POINT ( 'NONE',  ( -23.68543856465402797, 7.999999999999996447, -4.000000000000000000 ) ) ;
#2120=DIRECTION ( 'NONE',  ( 1.000000000000000000, 0.000000000000000000, 0.000000000000000000 ) ) ;
#2124=CARTESIAN_POINT ( 'NONE',  ( -16.10609822396473945, -5.439999999999995062, -4.000000000000000000 ) ) ;
#2125=VECTOR ( 'NONE', #175, 1000.000000000000114 ) ;
#2132=ADVANCED_FACE ( 'NONE', ( #1223 ), #2399, .F. ) ;
#2134=DIRECTION ( 'NONE',  ( 0.9474175425861609545, -0.3199999999999996181, 0.000000000000000000 ) ) ;
#2138=VERTEX_POINT ( 'NONE', #2375 ) ;
#2140=EDGE_CURVE ( 'NONE', #1912, #3903, #3472, .T. ) ;
#2141=DIRECTION ( 'NONE',  ( 0.000000000000000000, 0.000000000000000000, -1.000000000000000000 ) ) ;
#2145=FACE_OUTER_BOUND ( 'NONE', #3876, .T. ) ;
#2147=LINE ( 'NONE', #1814, #3952 ) ;
#2158=ORIENTED_EDGE ( 'NONE', *, *, #4675, .F. ) ;
#2161=EDGE_CURVE ( 'NONE', #2782, #2138, #4694, .T. ) ;
#2162=DIRECTION ( 'NONE',  ( 1.357798298438996130E-15, -1.000000000000000000, 0.000000000000000000 ) ) ;
#2163=CARTESIAN_POINT ( 'NONE',  ( 0.000000000000000000, 0.000000000000000000, -32.00000000000000000 ) ) ;
#2167=EDGE_CURVE ( 'NONE', #1558, #4122, #1305, .T. ) ;
#2175=CARTESIAN_POINT ( 'NONE',  ( -6.708203932499366751, -2.000000000000003553, -12.00000000000000000 ) ) ;
#2176=VECTOR ( 'NONE', #195, 1000.000000000000114 ) ;
#2177=DIRECTION ( 'NONE',  ( 1.000000000000000000, -0.000000000000000000, -0.000000000000000000 ) ) ;
#2178=AXIS2_PLACEMENT_3D ( 'NONE', #757, #267, #3364 ) ;
#2184=ORIENTED_EDGE ( 'NONE', *, *, #2530, .F. ) ;
#2185=VECTOR ( 'NONE', #4623, 1000.000000000000000 ) ;
#2191=ORIENTED_EDGE ( 'NONE', *, *, #3897, .F. ) ;
#2195=ORIENTED_EDGE ( 'NONE', *, *, #2530, .T. ) ;
#2199=CIRCLE ( 'NONE', #498, 6.999999999999999112 ) ;
#2201=CARTESIAN_POINT ( 'NONE',  ( 0.000000000000000000, 0.000000000000000000, 14.30577747056276472 ) ) ;
#2202=STYLED_ITEM ( 'NONE', ( #2298 ), #425 ) ;
#2215=CARTESIAN_POINT ( 'NONE',  ( -9.000000000000001776, 2.000000000000000000, -32.00000000000000000 ) ) ;
#2220=VERTEX_POINT ( 'NONE', #2897 ) ;
#2225=ADVANCED_FACE ( 'NONE', ( #3688 ), #4891, .F. ) ;
#2228=CARTESIAN_POINT ( 'NONE',  ( 0.000000000000000000, 0.000000000000000000, -4.000000000000000000 ) ) ;
#2236=AXIS2_PLACEMENT_3D ( 'NONE', #3594, #897, #3974 ) ;
#2248=UNCERTAINTY_MEASURE_WITH_UNIT (LENGTH_MEASURE( 1.000000000000000082E-05 ), #695, 'distance_accuracy_value', 'NONE');
#2249=DIRECTION ( 'NONE',  ( 0.000000000000000000, 0.000000000000000000, -1.000000000000000000 ) ) ;
#2258=FACE_OUTER_BOUND ( 'NONE', #1672, .T. ) ;
#2260=CARTESIAN_POINT ( 'NONE',  ( -6.517431832507181422E-14, 16.00000000000000000, -26.00000000000000355 ) ) ;
#2265=DIRECTION ( 'NONE',  ( -0.000000000000000000, -0.000000000000000000, 1.000000000000000000 ) ) ;
#2268=ORIENTED_EDGE ( 'NONE', *, *, #1447, .T. ) ;
#2273=VERTEX_POINT ( 'NONE', #2124 ) ;
#2275=FACE_OUTER_BOUND ( 'NONE', #1038, .T. ) ;
#2279=ORIENTED_EDGE ( 'NONE', *, *, #3940, .T. ) ;
#2290=CARTESIAN_POINT ( 'NONE',  ( -9.000000000000003553, -1.999999999999999112, -20.00000000000000000 ) ) ;
#2296=ORIENTED_EDGE ( 'NONE', *, *, #462, .T. ) ;
#2298=PRESENTATION_STYLE_ASSIGNMENT (( #4935 ) ) ;
#2300=ORIENTED_EDGE ( 'NONE', *, *, #2651, .T. ) ;
#2302=LINE ( 'NONE', #3751, #1857 ) ;
#2305=EDGE_CURVE ( 'NONE', #2020, #991, #269, .T. ) ;
#2309=EDGE_CURVE ( 'NONE', #4716, #536, #4752, .T. ) ;
#2315=EDGE_CURVE ( 'NONE', #1031, #4739, #171, .T. ) ;
#2316=EDGE_CURVE ( 'NONE', #148, #597, #2860, .T. ) ;
#2329=ORIENTED_EDGE ( 'NONE', *, *, #2349, .T. ) ;
#2334=DIRECTION ( 'NONE',  ( 0.000000000000000000, 0.000000000000000000, -1.000000000000000000 ) ) ;
#2343=AXIS2_PLACEMENT_3D ( 'NONE', #2260, #378, #3802 ) ;
#2347=ORIENTED_EDGE ( 'NONE', *, *, #4768, .F. ) ;
#2349=EDGE_CURVE ( 'NONE', #4716, #3536, #253, .T. ) ;
#2352=DIRECTION ( 'NONE',  ( 0.000000000000000000, 0.000000000000000000, -1.000000000000000000 ) ) ;
#2356=UNCERTAINTY_MEASURE_WITH_UNIT (LENGTH_MEASURE( 1.000000000000000082E-05 ), #630, 'distance_accuracy_value', 'NONE');
#2357=DIRECTION ( 'NONE',  ( 1.000000000000000000, 0.000000000000000000, 0.000000000000000000 ) ) ;
#2358=ADVANCED_FACE ( 'NONE', ( #1087 ), #2619, .T. ) ;
#2375=CARTESIAN_POINT ( 'NONE',  ( 0.000000000000000000, -25.00000000000000000, -20.00000000000000000 ) ) ;
#2396=VERTEX_POINT ( 'NONE', #336 ) ;
#2397=FILL_AREA_STYLE_COLOUR ( '', #1188 ) ;
#2399=CYLINDRICAL_SURFACE ( 'NONE', #1227, 2.099999999999997868 ) ;
#2401=CARTESIAN_POINT ( 'NONE',  ( 0.000000000000000000, 0.000000000000000000, -4.000000000000000000 ) ) ;
#2410=DIRECTION ( 'NONE',  ( 0.000000000000000000, 0.000000000000000000, -1.000000000000000000 ) ) ;
#2411=FACE_BOUND ( 'NONE', #3917, .T. ) ;
#2415=ORIENTED_EDGE ( 'NONE', *, *, #2349, .F. ) ;
#2417=AXIS2_PLACEMENT_3D ( 'NONE', #1786, #546, #1690 ) ;
#2426=AXIS2_PLACEMENT_3D ( 'NONE', #4042, #144, #4373 ) ;
#2427=VECTOR ( 'NONE', #561, 1000.000000000000000 ) ;
#2435=AXIS2_PLACEMENT_3D ( 'NONE', #4940, #2663, #2458 ) ;
#2437=EDGE_CURVE ( 'NONE', #4655, #4738, #2639, .T. ) ;
#2442=ORIENTED_EDGE ( 'NONE', *, *, #2309, .F. ) ;
#2457=CARTESIAN_POINT ( 'NONE',  ( -23.68543856465402442, -8.000000000000003553, -4.000000000000000000 ) ) ;
#2458=DIRECTION ( 'NONE',  ( -1.000000000000000000, 0.000000000000000000, 0.000000000000000000 ) ) ;
#2460=ORIENTED_EDGE ( 'NONE', *, *, #2010, .T. ) ;
#2461=ORIENTED_EDGE ( 'NONE', *, *, #4083, .F. ) ;
#2465=ADVANCED_FACE ( 'NONE', ( #4186 ), #758, .F. ) ;
#2469=DIRECTION ( 'NONE',  ( 1.000000000000000000, -0.000000000000000000, -0.000000000000000000 ) ) ;
#2470=DIRECTION ( 'NONE',  ( -0.000000000000000000, -0.000000000000000000, 1.000000000000000000 ) ) ;
#2476=CARTESIAN_POINT ( 'NONE',  ( 16.10609822396473589, 5.440000000000003055, -12.00000000000000000 ) ) ;
#2483=CARTESIAN_POINT ( 'NONE',  ( 0.000000000000000000, -1.999999999999999112, -12.00000000000000000 ) ) ;
#2485=CIRCLE ( 'NONE', #4962, 25.00000000000000000 ) ;
#2486=CARTESIAN_POINT ( 'NONE',  ( -16.10609822396473589, 5.440000000000003055, 14.30577747056276472 ) ) ;
#2492=EDGE_CURVE ( 'NONE', #4739, #4372, #495, .T. ) ;
#2496=ORIENTED_EDGE ( 'NONE', *, *, #288, .T. ) ;
#2504=LINE ( 'NONE', #551, #720 ) ;
#2506=AXIS2_PLACEMENT_3D ( 'NONE', #4, #1215, #4159 ) ;
#2507=VECTOR ( 'NONE', #3159, 1000.000000000000000 ) ;
#2509=EDGE_CURVE ( 'NONE', #654, #2138, #3564, .T. ) ;
#2512=DIRECTION ( 'NONE',  ( 1.000000000000000000, -0.000000000000000000, -0.000000000000000000 ) ) ;
#2517=FACE_OUTER_BOUND ( 'NONE', #4110, .T. ) ;
#2518=ORIENTED_EDGE ( 'NONE', *, *, #1051, .T. ) ;
#2521=LINE ( 'NONE', #2830, #2011 ) ;
#2527=DIRECTION ( 'NONE',  ( -1.000000000000000000, 0.000000000000000000, 0.000000000000000000 ) ) ;
#2530=EDGE_CURVE ( 'NONE', #2273, #121, #3543, .T. ) ;
#2532=LINE ( 'NONE', #2114, #2125 ) ;
#2533=ADVANCED_FACE ( 'NONE', ( #3889 ), #3913, .T. ) ;
#2541=FACE_OUTER_BOUND ( 'NONE', #3135, .T. ) ;
#2557=FACE_OUTER_BOUND ( 'NONE', #1266, .T. ) ;
#2572=VECTOR ( 'NONE', #3148, 1000.000000000000114 ) ;
#2573=CARTESIAN_POINT ( 'NONE',  ( 6.999999999999999112, 0.000000000000000000, -20.00000000000000000 ) ) ;
#2581=AXIS2_PLACEMENT_3D ( 'NONE', #112, #2823, #2120 ) ;
#2583=ORIENTED_EDGE ( 'NONE', *, *, #2305, .T. ) ;
#2586=AXIS2_PLACEMENT_3D ( 'NONE', #4358, #150, #1630 ) ;
#2593=AXIS2_PLACEMENT_3D ( 'NONE', #1909, #3047, #1562 ) ;
#2606=DIRECTION ( 'NONE',  ( 0.000000000000000000, 0.000000000000000000, -1.000000000000000000 ) ) ;
#2610=EDGE_CURVE ( 'NONE', #4618, #4395, #3492, .T. ) ;
#2614=CARTESIAN_POINT ( 'NONE',  ( -23.68543856465402797, 7.999999999999996447, 14.30577747056276472 ) ) ;
#2619=PLANE ( 'NONE',  #659 ) ;
#2638=CARTESIAN_POINT ( 'NONE',  ( -23.68543856465402797, 7.999999999999996447, -12.00000000000000000 ) ) ;
#2639=LINE ( 'NONE', #2290, #1691 ) ;
#2642=ORIENTED_EDGE ( 'NONE', *, *, #3742, .F. ) ;
#2643=EDGE_CURVE ( 'NONE', #9, #4655, #3222, .T. ) ;
#2650=ORIENTED_EDGE ( 'NONE', *, *, #174, .T. ) ;
#2651=EDGE_CURVE ( 'NONE', #537, #4618, #1368, .T. ) ;
#2654=LINE ( 'NONE', #3060, #236 ) ;
#2657=ORIENTED_EDGE ( 'NONE', *, *, #4083, .T. ) ;
#2663=DIRECTION ( 'NONE',  ( 0.000000000000000000, 0.000000000000000000, -1.000000000000000000 ) ) ;
#2670=CARTESIAN_POINT ( 'NONE',  ( 0.000000000000000000, 0.000000000000000000, -12.00000000000000000 ) ) ;
#2679=DIRECTION ( 'NONE',  ( 0.000000000000000000, 0.000000000000000000, 1.000000000000000000 ) ) ;
#2680=ORIENTED_EDGE ( 'NONE', *, *, #3940, .F. ) ;
#2686=ORIENTED_EDGE ( 'NONE', *, *, #3151, .F. ) ;
#2691=CYLINDRICAL_SURFACE ( 'NONE', #2343, 2.099999999999997868 ) ;
#2700=DIRECTION ( 'NONE',  ( 0.000000000000000000, 0.000000000000000000, 1.000000000000000000 ) ) ;
#2701=DIRECTION ( 'NONE',  ( 1.000000000000000000, -0.000000000000000000, -0.000000000000000000 ) ) ;
#2706=DIRECTION ( 'NONE',  ( 1.000000000000000000, 0.000000000000000000, 0.000000000000000000 ) ) ;
#2712=FACE_OUTER_BOUND ( 'NONE', #48, .T. ) ;
#2743=VECTOR ( 'NONE', #2067, 1000.000000000000000 ) ;
#2751=EDGE_CURVE ( 'NONE', #865, #536, #815, .T. ) ;
#2761=AXIS2_PLACEMENT_3D ( 'NONE', #4040, #3394, #611 ) ;
#2774=DIRECTION ( 'NONE',  ( 0.000000000000000000, 0.000000000000000000, -1.000000000000000000 ) ) ;
#2778=DIRECTION ( 'NONE',  ( -0.000000000000000000, -0.000000000000000000, -1.000000000000000000 ) ) ;
#2782=VERTEX_POINT ( 'NONE', #3679 ) ;
#2789=DIRECTION ( 'NONE',  ( 0.000000000000000000, 0.000000000000000000, -1.000000000000000000 ) ) ;
#2804=ORIENTED_EDGE ( 'NONE', *, *, #3153, .F. ) ;
#2822=DIRECTION ( 'NONE',  ( -0.000000000000000000, -0.000000000000000000, 1.000000000000000000 ) ) ;
#2823=DIRECTION ( 'NONE',  ( -0.000000000000000000, -0.000000000000000000, 1.000000000000000000 ) ) ;
#2824=AXIS2_PLACEMENT_3D ( 'NONE', #2163, #2822, #4814 ) ;
#2825=AXIS2_PLACEMENT_3D ( 'NONE', #1079, #3780, #2162 ) ;
#2829=VECTOR ( 'NONE', #3337, 1000.000000000000000 ) ;
#2830=CARTESIAN_POINT ( 'NONE',  ( -23.68543856465402797, 7.999999999999996447, 14.30577747056276472 ) ) ;
#2834=VERTEX_POINT ( 'NONE', #724 ) ;
#2844=DIRECTION ( 'NONE',  ( -1.000000000000000000, 0.000000000000000000, 0.000000000000000000 ) ) ;
#2847=DIRECTION ( 'NONE',  ( 0.000000000000000000, 0.000000000000000000, -1.000000000000000000 ) ) ;
#2857=ORIENTED_EDGE ( 'NONE', *, *, #3897, .T. ) ;
#2860=LINE ( 'NONE', #565, #2176 ) ;
#2869=ORIENTED_EDGE ( 'NONE', *, *, #800, .T. ) ;
#2881=DIRECTION ( 'NONE',  ( 1.000000000000000000, 0.000000000000000000, 0.000000000000000000 ) ) ;
#2896=PRODUCT_DEFINITION ( 'UNKNOWN', '', #4064, #3238 ) ;
#2897=CARTESIAN_POINT ( 'NONE',  ( -15.26180729995780716, -16.00000000000000355, -26.00000000000000355 ) ) ;
#2900=DIRECTION ( 'NONE',  ( -1.000000000000000000, 4.336808689942018722E-16, 0.000000000000000000 ) ) ;
#2901=AXIS2_PLACEMENT_3D ( 'NONE', #2071, #2097, #161 ) ;
#2903=VECTOR ( 'NONE', #2334, 1000.000000000000000 ) ;
#2908=AXIS2_PLACEMENT_3D ( 'NONE', #4178, #1960, #1879 ) ;
#2911=CARTESIAN_POINT ( 'NONE',  ( -23.68543856465402442, -8.000000000000003553, 14.30577747056276472 ) ) ;
#2921=DIRECTION ( 'NONE',  ( -1.000000000000000000, 0.000000000000000000, 0.000000000000000000 ) ) ;
#2925=ORIENTED_EDGE ( 'NONE', *, *, #288, .F. ) ;
#2931=LINE ( 'NONE', #1000, #4226 ) ;
#2947=ORIENTED_EDGE ( 'NONE', *, *, #2167, .F. ) ;
#2955=LINE ( 'NONE', #573, #4274 ) ;
#2977=VECTOR ( 'NONE', #1264, 1000.000000000000000 ) ;
#2979=VECTOR ( 'NONE', #2265, 1000.000000000000000 ) ;
#2985=FACE_OUTER_BOUND ( 'NONE', #4652, .T. ) ;
#2986=CIRCLE ( 'NONE', #2426, 2.099999999999997868 ) ;
#2989=DIRECTION ( 'NONE',  ( 0.000000000000000000, 0.000000000000000000, -1.000000000000000000 ) ) ;
#3000=CARTESIAN_POINT ( 'NONE',  ( -7.332110811570578784E-14, -6.999999999999999112, -32.00000000000000000 ) ) ;
#3001=DIRECTION ( 'NONE',  ( 2.168404344971009361E-16, -1.000000000000000000, 0.000000000000000000 ) ) ;
#3004=ORIENTED_EDGE ( 'NONE', *, *, #2315, .F. ) ;
#3005=FACE_OUTER_BOUND ( 'NONE', #4754, .T. ) ;
#3009=CARTESIAN_POINT ( 'NONE',  ( -6.537332342993324937E-14, 16.00000000000000000, -23.90000000000000568 ) ) ;
#3015=DIRECTION ( 'NONE',  ( 1.357798298438996130E-15, -1.000000000000000000, 0.000000000000000000 ) ) ;
#3032=EDGE_LOOP ( 'NONE', ( #491, #3733, #2857, #95 ) ) ;
#3044=VECTOR ( 'NONE', #1697, 1000.000000000000000 ) ;
#3047=DIRECTION ( 'NONE',  ( 0.000000000000000000, 0.000000000000000000, -1.000000000000000000 ) ) ;
#3054=CARTESIAN_POINT ( 'NONE',  ( -25.00000000000000000, 3.061616997868383043E-15, -32.00000000000000000 ) ) ;
#3056=ORIENTED_EDGE ( 'NONE', *, *, #2492, .F. ) ;
#3059=EDGE_CURVE ( 'NONE', #4410, #4395, #3509, .T. ) ;
#3060=CARTESIAN_POINT ( 'NONE',  ( -6.517431832507181422E-14, 16.00000000000000000, -23.90000000000000568 ) ) ;
#3061=EDGE_LOOP ( 'NONE', ( #4214, #143, #2461, #3886 ) ) ;
#3070=CARTESIAN_POINT ( 'NONE',  ( 23.68543856465402442, 7.999999999999994671, -12.00000000000000000 ) ) ;
#3077=DIRECTION ( 'NONE',  ( 1.000000000000000000, -0.000000000000000000, -0.000000000000000000 ) ) ;
#3078=FACE_BOUND ( 'NONE', #2109, .T. ) ;
#3080=CIRCLE ( 'NONE', #3701, 2.099999999999997868 ) ;
#3085=ORIENTED_EDGE ( 'NONE', *, *, #4424, .T. ) ;
#3088=DIRECTION ( 'NONE',  ( -0.000000000000000000, -0.000000000000000000, 1.000000000000000000 ) ) ;
#3095=CARTESIAN_POINT ( 'NONE',  ( -9.000000000000001776, 2.000000000000000000, -12.00000000000000000 ) ) ;
#3096=ORIENTED_EDGE ( 'NONE', *, *, #2309, .T. ) ;
#3124=ORIENTED_EDGE ( 'NONE', *, *, #4220, .F. ) ;
#3125=CIRCLE ( 'NONE', #242, 6.999999999999999112 ) ;
#3131=ORIENTED_EDGE ( 'NONE', *, *, #1669, .F. ) ;
#3132=DIRECTION ( 'NONE',  ( -1.000000000000000000, 0.000000000000000000, 0.000000000000000000 ) ) ;
#3135=EDGE_LOOP ( 'NONE', ( #4453, #2027, #2034, #2070, #2296, #2279 ) ) ;
#3148=DIRECTION ( 'NONE',  ( 0.9474175425861609545, 0.3199999999999996181, 0.000000000000000000 ) ) ;
#3151=EDGE_CURVE ( 'NONE', #4738, #4892, #151, .T. ) ;
#3153=EDGE_CURVE ( 'NONE', #1203, #4122, #910, .T. ) ;
#3157=SURFACE_STYLE_USAGE ( .BOTH. , #1614 ) ;
#3159=DIRECTION ( 'NONE',  ( -0.000000000000000000, -0.000000000000000000, 1.000000000000000000 ) ) ;
#3169=VECTOR ( 'NONE', #554, 1000.000000000000114 ) ;
#3173=ORIENTED_EDGE ( 'NONE', *, *, #2492, .T. ) ;
#3177=LINE ( 'NONE', #3634, #901 ) ;
#3179=ORIENTED_EDGE ( 'NONE', *, *, #3682, .T. ) ;
#3181=EDGE_CURVE ( 'NONE', #479, #2834, #2986, .T. ) ;
#3187=DIRECTION ( 'NONE',  ( -1.000000000000000000, 0.000000000000000000, 0.000000000000000000 ) ) ;
#3188=ORIENTED_EDGE ( 'NONE', *, *, #1884, .T. ) ;
#3190=ORIENTED_EDGE ( 'NONE', *, *, #4855, .T. ) ;
#3198=DIRECTION ( 'NONE',  ( 0.000000000000000000, 0.000000000000000000, -1.000000000000000000 ) ) ;
#3202=ORIENTED_EDGE ( 'NONE', *, *, #1910, .T. ) ;
#3208=AXIS2_PLACEMENT_3D ( 'NONE', #217, #1794, #4852 ) ;
#3214=DIRECTION ( 'NONE',  ( -1.000000000000000000, 0.000000000000000000, 0.000000000000000000 ) ) ;
#3222=LINE ( 'NONE', #3655, #2743 ) ;
#3223=DIRECTION ( 'NONE',  ( -0.3199999999999996736, 0.9474175425861610655, 0.000000000000000000 ) ) ;
#3238=PRODUCT_DEFINITION_CONTEXT ( 'detailed design', #1377, 'design' ) ;
#3260=DIRECTION ( 'NONE',  ( 0.000000000000000000, 0.000000000000000000, -1.000000000000000000 ) ) ;
#3270=ORIENTED_EDGE ( 'NONE', *, *, #2010, .F. ) ;
#3288=AXIS2_PLACEMENT_3D ( 'NONE', #1293, #2469, #194 ) ;
#3294=CYLINDRICAL_SURFACE ( 'NONE', #4103, 2.099999999999997868 ) ;
#3304=ADVANCED_FACE ( 'NONE', ( #344 ), #1412, .F. ) ;
#3307=ORIENTED_EDGE ( 'NONE', *, *, #323, .F. ) ;
#3322=CARTESIAN_POINT ( 'NONE',  ( 0.000000000000000000, 25.00000000000000000, -20.00000000000000000 ) ) ;
#3326=DIRECTION ( 'NONE',  ( -1.000000000000000000, 0.000000000000000000, 0.000000000000000000 ) ) ;
#3328=ORIENTED_EDGE ( 'NONE', *, *, #1162, .T. ) ;
#3332=CARTESIAN_POINT ( 'NONE',  ( -14.00000000000006395, 16.00000000000000000, -28.10000000000000142 ) ) ;
#3333=ORIENTED_EDGE ( 'NONE', *, *, #4943, .F. ) ;
#3337=DIRECTION ( 'NONE',  ( 0.5150380749100544886, 1.049727191138618449E-16, 0.8571673007021121116 ) ) ;
#3339=SHAPE_REPRESENTATION_RELATIONSHIP ( 'NONE' , 'NONE' ,  #3720, #469 ) ;
#3348=ORIENTED_EDGE ( 'NONE', *, *, #2167, .T. ) ;
#3351=SURFACE_SIDE_STYLE ('',( #353 ) ) ;
#3364=DIRECTION ( 'NONE',  ( 0.000000000000000000, 0.000000000000000000, -1.000000000000000000 ) ) ;
#3366=CARTESIAN_POINT ( 'NONE',  ( 6.517431832507181422E-14, -16.00000000000000000, -26.00000000000000355 ) ) ;
#3377=DIRECTION ( 'NONE',  ( 1.000000000000000000, -0.000000000000000000, -0.000000000000000000 ) ) ;
#3392=FACE_OUTER_BOUND ( 'NONE', #1760, .T. ) ;
#3394=DIRECTION ( 'NONE',  ( 0.000000000000000000, 0.000000000000000000, -1.000000000000000000 ) ) ;
#3395=ORIENTED_EDGE ( 'NONE', *, *, #2437, .F. ) ;
#3400=CARTESIAN_POINT ( 'NONE',  ( 0.000000000000000000, 0.000000000000000000, -4.000000000000000000 ) ) ;
#3409=DIRECTION ( 'NONE',  ( 0.9474175425861605104, -0.3200000000000010059, 0.000000000000000000 ) ) ;
#3410=VERTEX_POINT ( 'NONE', #1929 ) ;
#3411=EDGE_CURVE ( 'NONE', #4618, #9, #2302, .T. ) ;
#3416=EDGE_CURVE ( 'NONE', #4259, #852, #100, .T. ) ;
#3418=ORIENTED_EDGE ( 'NONE', *, *, #4481, .T. ) ;
#3423=STYLED_ITEM ( 'NONE', ( #3918 ), #469 ) ;
#3424=ORIENTED_EDGE ( 'NONE', *, *, #1027, .F. ) ;
#3433=AXIS2_PLACEMENT_3D ( 'NONE', #4374, #1647, #2881 ) ;
#3460=AXIS2_PLACEMENT_3D ( 'NONE', #1341, #238, #962 ) ;
#3465=ORIENTED_EDGE ( 'NONE', *, *, #1120, .F. ) ;
#3466=CIRCLE ( 'NONE', #2506, 17.00000000000000000 ) ;
#3467=ADVANCED_FACE ( 'NONE', ( #26 ), #1555, .T. ) ;
#3472=LINE ( 'NONE', #3920, #4823 ) ;
#3478=ADVANCED_FACE ( 'NONE', ( #2258 ), #3782, .F. ) ;
#3483=ORIENTED_EDGE ( 'NONE', *, *, #2316, .T. ) ;
#3484=ADVANCED_FACE ( 'NONE', ( #2411, #3905 ), #3559, .F. ) ;
#3492=LINE ( 'NONE', #3943, #4004 ) ;
#3496=LINE ( 'NONE', #1969, #4242 ) ;
#3498=DIRECTION ( 'NONE',  ( -1.000000000000000000, 0.000000000000000000, 0.000000000000000000 ) ) ;
#3502=ORIENTED_EDGE ( 'NONE', *, *, #4768, .T. ) ;
#3503=ORIENTED_EDGE ( 'NONE', *, *, #3648, .T. ) ;
#3509=LINE ( 'NONE', #1599, #4331 ) ;
#3513=CARTESIAN_POINT ( 'NONE',  ( -16.10609822396473945, -5.439999999999995062, 14.30577747056276472 ) ) ;
#3515=ORIENTED_EDGE ( 'NONE', *, *, #3411, .F. ) ;
#3518=DIRECTION ( 'NONE',  ( 1.000000000000000000, -7.105427357601001859E-15, 0.000000000000000000 ) ) ;
#3522=LINE ( 'NONE', #4352, #3044 ) ;
#3534=CARTESIAN_POINT ( 'NONE',  ( -14.00000000000006395, 16.00000000000000000, -23.90000000000000568 ) ) ;
#3536=VERTEX_POINT ( 'NONE', #3534 ) ;
#3537=ORIENTED_EDGE ( 'NONE', *, *, #4639, .F. ) ;
#3543=LINE ( 'NONE', #3513, #809 ) ;
#3559=PLANE ( 'NONE',  #2586 ) ;
#3564=LINE ( 'NONE', #1583, #2977 ) ;
#3576=CARTESIAN_POINT ( 'NONE',  ( 2.444036937190193033E-14, 6.999999999999999112, -32.00000000000000000 ) ) ;
#3587=EDGE_LOOP ( 'NONE', ( #3179, #4284, #3502, #2300, #1355, #782, #4387, #84, #4577 ) ) ;
#3589=DIRECTION ( 'NONE',  ( 1.000000000000000000, -0.000000000000000000, -0.000000000000000000 ) ) ;
#3594=CARTESIAN_POINT ( 'NONE',  ( 0.000000000000000000, 0.000000000000000000, -4.000000000000000000 ) ) ;
#3595=CARTESIAN_POINT ( 'NONE',  ( -14.00000000000006395, 16.00000000000000000, -26.00000000000000355 ) ) ;
#3608=DIRECTION ( 'NONE',  ( -0.9474175425861605104, -0.3200000000000010059, 0.000000000000000000 ) ) ;
#3616=DIRECTION ( 'NONE',  ( 1.000000000000000000, -0.000000000000000000, -0.000000000000000000 ) ) ;
#3619=CIRCLE ( 'NONE', #1457, 25.00000000000000000 ) ;
#3626=DIRECTION ( 'NONE',  ( 0.000000000000000000, 0.000000000000000000, -1.000000000000000000 ) ) ;
#3634=CARTESIAN_POINT ( 'NONE',  ( -13.99999999999993250, -16.00000000000000000, -28.10000000000000142 ) ) ;
#3636=ORIENTED_EDGE ( 'NONE', *, *, #2140, .T. ) ;
#3640=VERTEX_POINT ( 'NONE', #3703 ) ;
#3643=LINE ( 'NONE', #1364, #2086 ) ;
#3646=LINE ( 'NONE', #4027, #1715 ) ;
#3648=EDGE_CURVE ( 'NONE', #4131, #4716, #1803, .T. ) ;
#3655=CARTESIAN_POINT ( 'NONE',  ( -9.000000000000001776, 2.000000000000000000, -32.00000000000000000 ) ) ;
#3658=ADVANCED_FACE ( 'NONE', ( #3844 ), #1173, .T. ) ;
#3660=LINE ( 'NONE', #4413, #4326 ) ;
#3664=CARTESIAN_POINT ( 'NONE',  ( -13.99999999999993250, -16.00000000000000000, -23.90000000000000568 ) ) ;
#3667=ORIENTED_EDGE ( 'NONE', *, *, #1645, .T. ) ;
#3677=CARTESIAN_POINT ( 'NONE',  ( 23.68543856465402797, 7.999999999999996447, -4.000000000000000000 ) ) ;
#3679=CARTESIAN_POINT ( 'NONE',  ( 0.000000000000000000, -25.00000000000000000, -32.00000000000000000 ) ) ;
#3682=EDGE_CURVE ( 'NONE', #2782, #2020, #3619, .T. ) ;
#3686=CARTESIAN_POINT ( 'NONE',  ( 6.999999999999999112, 0.000000000000000000, -12.00000000000000000 ) ) ;
#3688=FACE_OUTER_BOUND ( 'NONE', #2008, .T. ) ;
#3697=DIRECTION ( 'NONE',  ( -0.000000000000000000, -0.000000000000000000, 1.000000000000000000 ) ) ;
#3698=DIRECTION ( 'NONE',  ( 0.000000000000000000, 0.000000000000000000, -1.000000000000000000 ) ) ;
#3701=AXIS2_PLACEMENT_3D ( 'NONE', #4349, #1389, #4870 ) ;
#3703=CARTESIAN_POINT ( 'NONE',  ( 25.00000000000000000, 0.000000000000000000, -20.00000000000000000 ) ) ;
#3709=EDGE_LOOP ( 'NONE', ( #2925, #969, #1775, #3667 ) ) ;
#3716=CARTESIAN_POINT ( 'NONE',  ( -14.00000000000006395, 16.00000000000000000, -26.00000000000000355 ) ) ;
#3720=SHAPE_REPRESENTATION ( 'Output Clamping Hub Sleeve', ( #1918 ), #4450 ) ;
#3721=EDGE_LOOP ( 'NONE', ( #3465, #4334, #2642, #977, #3307, #4257 ) ) ;
#3723=LINE ( 'NONE', #593, #3998 ) ;
#3729=ORIENTED_EDGE ( 'NONE', *, *, #4261, .T. ) ;
#3733=ORIENTED_EDGE ( 'NONE', *, *, #1182, .T. ) ;
#3742=EDGE_CURVE ( 'NONE', #4175, #2273, #518, .T. ) ;
#3751=CARTESIAN_POINT ( 'NONE',  ( -9.000000000000001776, 2.000000000000000000, -32.00000000000000000 ) ) ;
#3753=CARTESIAN_POINT ( 'NONE',  ( 23.68543856465402442, -8.000000000000003553, 14.30577747056276472 ) ) ;
#3762=AXIS2_PLACEMENT_3D ( 'NONE', #3842, #2778, #4211 ) ;
#3775=VECTOR ( 'NONE', #1729, 1000.000000000000000 ) ;
#3780=DIRECTION ( 'NONE',  ( -1.000000000000000000, -1.357798298438996130E-15, 0.000000000000000000 ) ) ;
#3782=CYLINDRICAL_SURFACE ( 'NONE', #2435, 17.00000000000000000 ) ;
#3786=ORIENTED_EDGE ( 'NONE', *, *, #4533, .F. ) ;
#3787=CARTESIAN_POINT ( 'NONE',  ( -13.99999999999993250, -16.00000000000000000, -28.10000000000000142 ) ) ;
#3796=CARTESIAN_POINT ( 'NONE',  ( 0.000000000000000000, 0.000000000000000000, -4.000000000000000000 ) ) ;
#3799=CARTESIAN_POINT ( 'NONE',  ( 23.68543856465402797, 7.999999999999996447, 14.30577747056276472 ) ) ;
#3800=DIRECTION ( 'NONE',  ( 0.000000000000000000, 0.000000000000000000, -1.000000000000000000 ) ) ;
#3802=DIRECTION ( 'NONE',  ( 0.000000000000000000, 0.000000000000000000, -1.000000000000000000 ) ) ;
#3828=EDGE_CURVE ( 'NONE', #597, #4842, #109, .T. ) ;
#3829=AXIS2_PLACEMENT_3D ( 'NONE', #4275, #1920, #2706 ) ;
#3842=CARTESIAN_POINT ( 'NONE',  ( 0.000000000000000000, 0.000000000000000000, -4.000000000000000000 ) ) ;
#3844=FACE_OUTER_BOUND ( 'NONE', #584, .T. ) ;
#3848=VECTOR ( 'NONE', #2470, 1000.000000000000000 ) ;
#3850=DIRECTION ( 'NONE',  ( 0.000000000000000000, 0.000000000000000000, 1.000000000000000000 ) ) ;
#3855=VECTOR ( 'NONE', #4783, 1000.000000000000000 ) ;
#3857=AXIS2_PLACEMENT_3D ( 'NONE', #951, #2512, #2410 ) ;
#3863=ORIENTED_EDGE ( 'NONE', *, *, #3925, .F. ) ;
#3876=EDGE_LOOP ( 'NONE', ( #3999, #3328, #2869 ) ) ;
#3878=ADVANCED_FACE ( 'NONE', ( #1735 ), #3921, .F. ) ;
#3882=ORIENTED_EDGE ( 'NONE', *, *, #3828, .T. ) ;
#3886=ORIENTED_EDGE ( 'NONE', *, *, #1645, .F. ) ;
#3889=FACE_OUTER_BOUND ( 'NONE', #4036, .T. ) ;
#3897=EDGE_CURVE ( 'NONE', #2834, #479, #3080, .T. ) ;
#3898=ORIENTED_EDGE ( 'NONE', *, *, #3416, .T. ) ;
#3899=CARTESIAN_POINT ( 'NONE',  ( 0.000000000000000000, 0.000000000000000000, -32.00000000000000000 ) ) ;
#3903=VERTEX_POINT ( 'NONE', #3322 ) ;
#3905=FACE_OUTER_BOUND ( 'NONE', #1083, .T. ) ;
#3911=SHAPE_DEFINITION_REPRESENTATION ( #1774, #3720 ) ;
#3913=CYLINDRICAL_SURFACE ( 'NONE', #413, 25.00000000000000000 ) ;
#3914=CARTESIAN_POINT ( 'NONE',  ( -9.000000000000003553, -1.999999999999999112, -32.00000000000000000 ) ) ;
#3917=EDGE_LOOP ( 'NONE', ( #4154, #2191 ) ) ;
#3918=PRESENTATION_STYLE_ASSIGNMENT (( #3157 ) ) ;
#3920=CARTESIAN_POINT ( 'NONE',  ( 0.000000000000000000, 25.00000000000000000, -32.00000000000000000 ) ) ;
#3921=PLANE ( 'NONE',  #279 ) ;
#3925=EDGE_CURVE ( 'NONE', #537, #4259, #2147, .T. ) ;
#3930=AXIS2_PLACEMENT_3D ( 'NONE', #2, #1035, #1531 ) ;
#3939=VECTOR ( 'NONE', #4786, 1000.000000000000000 ) ;
#3940=EDGE_CURVE ( 'NONE', #3640, #2138, #1783, .T. ) ;
#3943=CARTESIAN_POINT ( 'NONE',  ( -6.708203932499367639, 2.000000000000000888, -20.00000000000000000 ) ) ;
#3944=CARTESIAN_POINT ( 'NONE',  ( -15.26180729995793861, 15.99999999999999645, -26.00000000000000355 ) ) ;
#3950=DIRECTION ( 'NONE',  ( -1.000000000000000000, 0.000000000000000000, 0.000000000000000000 ) ) ;
#3952=VECTOR ( 'NONE', #4485, 1000.000000000000000 ) ;
#3965=DIRECTION ( 'NONE',  ( 1.000000000000000000, -0.000000000000000000, -0.000000000000000000 ) ) ;
#3970=CARTESIAN_POINT ( 'NONE',  ( -6.708203932499366751, -2.000000000000003553, -32.00000000000000000 ) ) ;
#3974=DIRECTION ( 'NONE',  ( 1.000000000000000000, 0.000000000000000000, 0.000000000000000000 ) ) ;
#3982=ORIENTED_EDGE ( 'NONE', *, *, #4911, .T. ) ;
#3990=ADVANCED_FACE ( 'NONE', ( #1757 ), #3294, .F. ) ;
#3993=VERTEX_POINT ( 'NONE', #4136 ) ;
#3998=VECTOR ( 'NONE', #3697, 1000.000000000000000 ) ;
#3999=ORIENTED_EDGE ( 'NONE', *, *, #3648, .F. ) ;
#4004=VECTOR ( 'NONE', #806, 1000.000000000000000 ) ;
#4010=ORIENTED_EDGE ( 'NONE', *, *, #1316, .F. ) ;
#4027=CARTESIAN_POINT ( 'NONE',  ( 1.387778780781444295E-15, 4.108768631691174362E-15, -12.00000000000000000 ) ) ;
#4031=AXIS2_PLACEMENT_3D ( 'NONE', #2670, #2789, #2844 ) ;
#4036=EDGE_LOOP ( 'NONE', ( #4010, #2583, #1914, #903, #3190, #1567, #4702, #509, #4227, #4408 ) ) ;
#4040=CARTESIAN_POINT ( 'NONE',  ( 0.000000000000000000, 0.000000000000000000, -20.00000000000000000 ) ) ;
#4042=CARTESIAN_POINT ( 'NONE',  ( 6.497531322021036645E-14, -16.00000000000000000, -26.00000000000000355 ) ) ;
#4047=FACE_OUTER_BOUND ( 'NONE', #911, .T. ) ;
#4060=CARTESIAN_POINT ( 'NONE',  ( -23.68543856465402442, -8.000000000000003553, -4.000000000000000000 ) ) ;
#4064=PRODUCT_DEFINITION_FORMATION_WITH_SPECIFIED_SOURCE ( 'ANY', '', #1016, .NOT_KNOWN. ) ;
#4068=ORIENTED_EDGE ( 'NONE', *, *, #2316, .F. ) ;
#4069=ADVANCED_FACE ( 'NONE', ( #3078, #58 ), #4534, .F. ) ;
#4077=AXIS2_PLACEMENT_3D ( 'NONE', #1171, #419, #3518 ) ;
#4082=CIRCLE ( 'NONE', #254, 25.00000000000000000 ) ;
#4083=EDGE_CURVE ( 'NONE', #3410, #811, #3466, .T. ) ;
#4103=AXIS2_PLACEMENT_3D ( 'NONE', #3366, #4896, #4826 ) ;
#4110=EDGE_LOOP ( 'NONE', ( #530, #3503, #2329 ) ) ;
#4119=CARTESIAN_POINT ( 'NONE',  ( 0.000000000000000000, 0.000000000000000000, -12.00000000000000000 ) ) ;
#4122=VERTEX_POINT ( 'NONE', #4385 ) ;
#4125=CARTESIAN_POINT ( 'NONE',  ( 0.000000000000000000, 0.000000000000000000, -4.000000000000000000 ) ) ;
#4128=CARTESIAN_POINT ( 'NONE',  ( 0.000000000000000000, 0.000000000000000000, -32.00000000000000000 ) ) ;
#4130=CARTESIAN_POINT ( 'NONE',  ( -13.99999999999993250, -16.00000000000000000, -23.90000000000000568 ) ) ;
#4131=VERTEX_POINT ( 'NONE', #3944 ) ;
#4132=EDGE_LOOP ( 'NONE', ( #3056, #4468, #3188, #4961 ) ) ;
#4136=CARTESIAN_POINT ( 'NONE',  ( 23.68543856465402797, 7.999999999999996447, -4.000000000000000000 ) ) ;
#4138=( GEOMETRIC_REPRESENTATION_CONTEXT ( 3 ) GLOBAL_UNCERTAINTY_ASSIGNED_CONTEXT ( ( #2356 ) ) GLOBAL_UNIT_ASSIGNED_CONTEXT ( ( #630, #265, #1810 ) ) REPRESENTATION_CONTEXT ( 'NONE', 'WORKASPACE' ) );
#4146=ADVANCED_FACE ( 'NONE', ( #1289 ), #4287, .T. ) ;
#4148=ORIENTED_EDGE ( 'NONE', *, *, #2161, .T. ) ;
#4149=AXIS2_PLACEMENT_3D ( 'NONE', #642, #4518, #2249 ) ;
#4153=DIRECTION ( 'NONE',  ( -0.9474175425861609545, 0.3199999999999996181, 0.000000000000000000 ) ) ;
#4154=ORIENTED_EDGE ( 'NONE', *, *, #3181, .F. ) ;
#4158=DIRECTION ( 'NONE',  ( 1.000000000000000000, 2.168404344971009361E-16, 0.000000000000000000 ) ) ;
#4159=DIRECTION ( 'NONE',  ( -1.000000000000000000, 0.000000000000000000, 0.000000000000000000 ) ) ;
#4171=AXIS2_PLACEMENT_3D ( 'NONE', #4478, #1781, #210 ) ;
#4173=EDGE_CURVE ( 'NONE', #4655, #1319, #937, .T. ) ;
#4174=EDGE_CURVE ( 'NONE', #121, #4122, #1244, .T. ) ;
#4175=VERTEX_POINT ( 'NONE', #4715 ) ;
#4178=CARTESIAN_POINT ( 'NONE',  ( 0.000000000000000000, 0.000000000000000000, -20.00000000000000000 ) ) ;
#4186=FACE_OUTER_BOUND ( 'NONE', #1455, .T. ) ;
#4190=ORIENTED_EDGE ( 'NONE', *, *, #2003, .F. ) ;
#4193=ORIENTED_EDGE ( 'NONE', *, *, #3925, .T. ) ;
#4196=ADVANCED_FACE ( 'NONE', ( #1336 ), #496, .F. ) ;
#4197=ORIENTED_EDGE ( 'NONE', *, *, #2161, .F. ) ;
#4202=DIRECTION ( 'NONE',  ( -0.3200000000000010614, -0.9474175425861606215, 0.000000000000000000 ) ) ;
#4207=DIRECTION ( 'NONE',  ( 1.000000000000000000, 0.000000000000000000, 0.000000000000000000 ) ) ;
#4211=DIRECTION ( 'NONE',  ( 1.000000000000000000, 3.552713678800500929E-15, 0.000000000000000000 ) ) ;
#4214=ORIENTED_EDGE ( 'NONE', *, *, #4608, .T. ) ;
#4216=CARTESIAN_POINT ( 'NONE',  ( 6.999999999999999112, 0.000000000000000000, -20.00000000000000000 ) ) ;
#4217=FILL_AREA_STYLE ('',( #1152 ) ) ;
#4220=EDGE_CURVE ( 'NONE', #2220, #1467, #3177, .T. ) ;
#4226=VECTOR ( 'NONE', #694, 1000.000000000000000 ) ;
#4227=ORIENTED_EDGE ( 'NONE', *, *, #462, .F. ) ;
#4235=EDGE_CURVE ( 'NONE', #4410, #4738, #984, .T. ) ;
#4237=CIRCLE ( 'NONE', #83, 2.099999999999997868 ) ;
#4239=CARTESIAN_POINT ( 'NONE',  ( -14.00000000000006395, 16.00000000000000000, -23.90000000000000568 ) ) ;
#4242=VECTOR ( 'NONE', #2701, 1000.000000000000000 ) ;
#4253=VECTOR ( 'NONE', #359, 1000.000000000000000 ) ;
#4257=ORIENTED_EDGE ( 'NONE', *, *, #4729, .F. ) ;
#4259=VERTEX_POINT ( 'NONE', #1451 ) ;
#4261=EDGE_CURVE ( 'NONE', #2220, #4937, #626, .T. ) ;
#4268=ORIENTED_EDGE ( 'NONE', *, *, #1669, .T. ) ;
#4274=VECTOR ( 'NONE', #3626, 1000.000000000000000 ) ;
#4275=CARTESIAN_POINT ( 'NONE',  ( 0.000000000000000000, 0.000000000000000000, -20.00000000000000000 ) ) ;
#4284=ORIENTED_EDGE ( 'NONE', *, *, #1316, .T. ) ;
#4287=PLANE ( 'NONE',  #579 ) ;
#4292=FILL_AREA_STYLE ('',( #2397 ) ) ;
#4305=ADVANCED_FACE ( 'NONE', ( #2517 ), #4487, .F. ) ;
#4314=CIRCLE ( 'NONE', #1118, 17.00000000000000000 ) ;
#4317=CIRCLE ( 'NONE', #1284, 17.00000000000000000 ) ;
#4319=CARTESIAN_POINT ( 'NONE',  ( 16.10609822396473945, -5.439999999999995062, -12.00000000000000000 ) ) ;
#4321=DIRECTION ( 'NONE',  ( -4.336808689942018722E-16, -1.000000000000000000, 0.000000000000000000 ) ) ;
#4324=DIRECTION ( 'NONE',  ( 0.000000000000000000, 0.000000000000000000, -1.000000000000000000 ) ) ;
#4326=VECTOR ( 'NONE', #3589, 1000.000000000000000 ) ;
#4331=VECTOR ( 'NONE', #1578, 1000.000000000000000 ) ;
#4334=ORIENTED_EDGE ( 'NONE', *, *, #196, .F. ) ;
#4344=ORIENTED_EDGE ( 'NONE', *, *, #4424, .F. ) ;
#4348=CARTESIAN_POINT ( 'NONE',  ( 0.000000000000000000, -25.00000000000000000, -32.00000000000000000 ) ) ;
#4349=CARTESIAN_POINT ( 'NONE',  ( 6.497531322021036645E-14, -16.00000000000000000, -26.00000000000000355 ) ) ;
#4352=CARTESIAN_POINT ( 'NONE',  ( 0.000000000000000000, 25.00000000000000000, -32.00000000000000000 ) ) ;
#4358=CARTESIAN_POINT ( 'NONE',  ( -7.332110811570578784E-14, -6.999999999999999112, -32.00000000000000000 ) ) ;
#4362=ADVANCED_FACE ( 'NONE', ( #1082 ), #1029, .T. ) ;
#4370=CARTESIAN_POINT ( 'NONE',  ( -25.00000000000000000, 3.061616997868383043E-15, -20.00000000000000000 ) ) ;
#4371=DIRECTION ( 'NONE',  ( 1.000000000000000000, 0.000000000000000000, 0.000000000000000000 ) ) ;
#4372=VERTEX_POINT ( 'NONE', #3070 ) ;
#4373=DIRECTION ( 'NONE',  ( 0.000000000000000000, 0.000000000000000000, -1.000000000000000000 ) ) ;
#4374=CARTESIAN_POINT ( 'NONE',  ( 0.000000000000000000, 0.000000000000000000, -4.000000000000000000 ) ) ;
#4383=CARTESIAN_POINT ( 'NONE',  ( -23.68543856465402797, 7.999999999999996447, -4.000000000000000000 ) ) ;
#4385=CARTESIAN_POINT ( 'NONE',  ( -23.68543856465402442, -8.000000000000003553, -12.00000000000000000 ) ) ;
#4387=ORIENTED_EDGE ( 'NONE', *, *, #4173, .T. ) ;
#4391=ADVANCED_FACE ( 'NONE', ( #2712 ), #2691, .F. ) ;
#4395=VERTEX_POINT ( 'NONE', #4553 ) ;
#4401=ADVANCED_FACE ( 'NONE', ( #3005 ), #4916, .T. ) ;
#4405=CARTESIAN_POINT ( 'NONE',  ( -9.000000000000001776, 3.903127820947817540E-15, -12.00000000000000000 ) ) ;
#4408=ORIENTED_EDGE ( 'NONE', *, *, #2140, .F. ) ;
#4410=VERTEX_POINT ( 'NONE', #3095 ) ;
#4413=CARTESIAN_POINT ( 'NONE',  ( 6.517431832507181422E-14, -16.00000000000000000, -23.90000000000000568 ) ) ;
#4424=EDGE_CURVE ( 'NONE', #1319, #4892, #1557, .T. ) ;
#4426=PLANE ( 'NONE',  #1058 ) ;
#4450=( GEOMETRIC_REPRESENTATION_CONTEXT ( 3 ) GLOBAL_UNCERTAINTY_ASSIGNED_CONTEXT ( ( #790 ) ) GLOBAL_UNIT_ASSIGNED_CONTEXT ( ( #921, #544, #474 ) ) REPRESENTATION_CONTEXT ( 'NONE', 'WORKASPACE' ) );
#4453=ORIENTED_EDGE ( 'NONE', *, *, #2509, .F. ) ;
#4468=ORIENTED_EDGE ( 'NONE', *, *, #4481, .F. ) ;
#4478=CARTESIAN_POINT ( 'NONE',  ( -14.00000000000006395, 16.00000000000000000, -26.00000000000000355 ) ) ;
#4481=EDGE_CURVE ( 'NONE', #4842, #4739, #2931, .T. ) ;
#4485=DIRECTION ( 'NONE',  ( -0.000000000000000000, -0.000000000000000000, 1.000000000000000000 ) ) ;
#4487=CONICAL_SURFACE ( 'NONE', #4171, 2.099999999999997868, 1.029744258676654090 ) ;
#4509=CARTESIAN_POINT ( 'NONE',  ( 25.00000000000000000, 0.000000000000000000, -4.000000000000000000 ) ) ;
#4516=CARTESIAN_POINT ( 'NONE',  ( -17.00000000000000000, 0.000000000000000000, -12.00000000000000000 ) ) ;
#4518=DIRECTION ( 'NONE',  ( 1.000000000000000000, -0.000000000000000000, -0.000000000000000000 ) ) ;
#4519=CARTESIAN_POINT ( 'NONE',  ( 0.000000000000000000, 0.000000000000000000, -20.00000000000000000 ) ) ;
#4524=CARTESIAN_POINT ( 'NONE',  ( 0.000000000000000000, 25.00000000000000000, -32.00000000000000000 ) ) ;
#4533=EDGE_CURVE ( 'NONE', #1467, #4937, #2081, .T. ) ;
#4534=PLANE ( 'NONE',  #2593 ) ;
#4540=ADVANCED_FACE ( 'NONE', ( #4047 ), #319, .T. ) ;
#4548=ORIENTED_EDGE ( 'NONE', *, *, #4174, .T. ) ;
#4553=CARTESIAN_POINT ( 'NONE',  ( -6.708203932499367639, 2.000000000000000888, -12.00000000000000000 ) ) ;
#4564=DIRECTION ( 'NONE',  ( 1.000000000000000000, 0.000000000000000000, 0.000000000000000000 ) ) ;
#4573=CYLINDRICAL_SURFACE ( 'NONE', #713, 17.00000000000000000 ) ;
#4577=ORIENTED_EDGE ( 'NONE', *, *, #708, .T. ) ;
#4578=EDGE_LOOP ( 'NONE', ( #4709, #3786, #2518, #1261 ) ) ;
#4581=CLOSED_SHELL ( 'NONE', ( #3990, #483, #4391, #1178, #4722, #3304, #2533, #4634, #1329, #4069, #1421, #3878, #2358, #4196, #4362, #4856, #4540, #2012, #4401, #3478, #4146, #3658, #1853, #3484, #3467, #4305, #2465, #2225, #2132 ) ) ;
#4584=DIRECTION ( 'NONE',  ( -1.000000000000000000, 0.000000000000000000, -0.000000000000000000 ) ) ;
#4592=CARTESIAN_POINT ( 'NONE',  ( 23.68543856465402442, -8.000000000000003553, -12.00000000000000000 ) ) ;
#4603=( NAMED_UNIT ( * ) SI_UNIT ( $, .STERADIAN. ) SOLID_ANGLE_UNIT ( ) );
#4607=EDGE_LOOP ( 'NONE', ( #3537, #460, #1436, #2158, #3085, #4710 ) ) ;
#4608=EDGE_CURVE ( 'NONE', #1339, #4175, #4314, .T. ) ;
#4611=CARTESIAN_POINT ( 'NONE',  ( -6.708203932499366751, -2.000000000000003553, -20.00000000000000000 ) ) ;
#4618=VERTEX_POINT ( 'NONE', #1872 ) ;
#4623=DIRECTION ( 'NONE',  ( 0.5150380749100544886, 0.000000000000000000, -0.8571673007021121116 ) ) ;
#4634=ADVANCED_FACE ( 'NONE', ( #2275 ), #1151, .T. ) ;
#4639=EDGE_CURVE ( 'NONE', #852, #54, #850, .T. ) ;
#4650=CARTESIAN_POINT ( 'NONE',  ( -14.00000000000006395, 16.00000000000000000, -28.10000000000000142 ) ) ;
#4651=CARTESIAN_POINT ( 'NONE',  ( -3.666055405785289392E-14, -6.999999999999999112, -20.00000000000000000 ) ) ;
#4652=EDGE_LOOP ( 'NONE', ( #3124, #3729, #1994 ) ) ;
#4655=VERTEX_POINT ( 'NONE', #4934 ) ;
#4663=ORIENTED_EDGE ( 'NONE', *, *, #4235, .F. ) ;
#4675=EDGE_CURVE ( 'NONE', #1319, #2396, #3125, .T. ) ;
#4694=LINE ( 'NONE', #4348, #2507 ) ;
#4702=ORIENTED_EDGE ( 'NONE', *, *, #1027, .T. ) ;
#4705=EDGE_CURVE ( 'NONE', #3536, #865, #2654, .T. ) ;
#4709=ORIENTED_EDGE ( 'NONE', *, *, #1182, .F. ) ;
#4710=ORIENTED_EDGE ( 'NONE', *, *, #1996, .F. ) ;
#4715=CARTESIAN_POINT ( 'NONE',  ( -17.00000000000000000, 0.000000000000000000, -4.000000000000000000 ) ) ;
#4716=VERTEX_POINT ( 'NONE', #4650 ) ;
#4722=ADVANCED_FACE ( 'NONE', ( #1228 ), #4573, .F. ) ;
#4729=EDGE_CURVE ( 'NONE', #991, #1722, #396, .T. ) ;
#4734=CARTESIAN_POINT ( 'NONE',  ( 7.216449660063538023E-15, 2.136559688479409280E-14, -12.00000000000000000 ) ) ;
#4738=VERTEX_POINT ( 'NONE', #927 ) ;
#4739=VERTEX_POINT ( 'NONE', #2476 ) ;
#4745=DIRECTION ( 'NONE',  ( -0.9474175425861609545, -0.3199999999999996181, 0.000000000000000000 ) ) ;
#4750=ORIENTED_EDGE ( 'NONE', *, *, #4174, .F. ) ;
#4752=LINE ( 'NONE', #633, #1441 ) ;
#4754=EDGE_LOOP ( 'NONE', ( #4190, #707, #3483, #4268 ) ) ;
#4768=EDGE_CURVE ( 'NONE', #1912, #537, #3522, .T. ) ;
#4774=ORIENTED_EDGE ( 'NONE', *, *, #3059, .F. ) ;
#4780=ORIENTED_EDGE ( 'NONE', *, *, #4785, .T. ) ;
#4783=DIRECTION ( 'NONE',  ( 1.000000000000000000, -0.000000000000000000, 0.000000000000000000 ) ) ;
#4785=EDGE_CURVE ( 'NONE', #1343, #148, #631, .T. ) ;
#4786=DIRECTION ( 'NONE',  ( 0.000000000000000000, 0.000000000000000000, -1.000000000000000000 ) ) ;
#4788=DIRECTION ( 'NONE',  ( 0.3199999999999996736, 0.9474175425861610655, 0.000000000000000000 ) ) ;
#4796=CARTESIAN_POINT ( 'NONE',  ( -9.000000000000001776, 3.903127820947817540E-15, -20.00000000000000000 ) ) ;
#4799=AXIS2_PLACEMENT_3D ( 'NONE', #2911, #4878, #351 ) ;
#4800=DIRECTION ( 'NONE',  ( -1.000000000000000000, 0.000000000000000000, 0.000000000000000000 ) ) ;
#4808=CONICAL_SURFACE ( 'NONE', #3288, 2.099999999999997868, 1.029744258676654090 ) ;
#4814=DIRECTION ( 'NONE',  ( -1.000000000000000000, 0.000000000000000000, 0.000000000000000000 ) ) ;
#4821=AXIS2_PLACEMENT_3D ( 'NONE', #2614, #4788, #4153 ) ;
#4822=CARTESIAN_POINT ( 'NONE',  ( 0.000000000000000000, 0.000000000000000000, -32.00000000000000000 ) ) ;
#4823=VECTOR ( 'NONE', #502, 1000.000000000000000 ) ;
#4826=DIRECTION ( 'NONE',  ( 0.000000000000000000, 0.000000000000000000, -1.000000000000000000 ) ) ;
#4831=DIRECTION ( 'NONE',  ( 0.000000000000000000, 0.000000000000000000, -1.000000000000000000 ) ) ;
#4842=VERTEX_POINT ( 'NONE', #689 ) ;
#4843=ORIENTED_EDGE ( 'NONE', *, *, #2651, .F. ) ;
#4851=DIRECTION ( 'NONE',  ( -0.000000000000000000, -0.000000000000000000, 1.000000000000000000 ) ) ;
#4852=DIRECTION ( 'NONE',  ( 0.000000000000000000, 0.000000000000000000, -1.000000000000000000 ) ) ;
#4854=ORIENTED_EDGE ( 'NONE', *, *, #4855, .F. ) ;
#4855=EDGE_CURVE ( 'NONE', #1390, #4372, #2485, .T. ) ;
#4856=ADVANCED_FACE ( 'NONE', ( #1433 ), #1017, .F. ) ;
#4870=DIRECTION ( 'NONE',  ( 0.000000000000000000, 0.000000000000000000, -1.000000000000000000 ) ) ;
#4871=ORIENTED_EDGE ( 'NONE', *, *, #2643, .F. ) ;
#4878=DIRECTION ( 'NONE',  ( 0.3200000000000010614, -0.9474175425861606215, 0.000000000000000000 ) ) ;
#4882=EDGE_CURVE ( 'NONE', #3640, #1343, #3643, .T. ) ;
#4885=FACE_BOUND ( 'NONE', #324, .T. ) ;
#4891=CONICAL_SURFACE ( 'NONE', #3460, 2.099999999999997868, 1.029744258676654090 ) ;
#4892=VERTEX_POINT ( 'NONE', #2175 ) ;
#4893=LINE ( 'NONE', #3000, #2979 ) ;
#4896=DIRECTION ( 'NONE',  ( 1.000000000000000000, -0.000000000000000000, -0.000000000000000000 ) ) ;
#4902=DIRECTION ( 'NONE',  ( -0.000000000000000000, -0.000000000000000000, 1.000000000000000000 ) ) ;
#4911=EDGE_CURVE ( 'NONE', #9, #4410, #3723, .T. ) ;
#4912=EDGE_CURVE ( 'NONE', #4937, #1467, #399, .T. ) ;
#4916=PLANE ( 'NONE',  #1376 ) ;
#4925=DIRECTION ( 'NONE',  ( 0.000000000000000000, 0.000000000000000000, -1.000000000000000000 ) ) ;
#4934=CARTESIAN_POINT ( 'NONE',  ( -9.000000000000003553, -1.999999999999999112, -32.00000000000000000 ) ) ;
#4935=SURFACE_STYLE_USAGE ( .BOTH. , #3351 ) ;
#4937=VERTEX_POINT ( 'NONE', #3664 ) ;
#4940=CARTESIAN_POINT ( 'NONE',  ( 0.000000000000000000, 0.000000000000000000, 14.30577747056276472 ) ) ;
#4943=EDGE_CURVE ( 'NONE', #811, #121, #4317, .T. ) ;
#4959=VECTOR ( 'NONE', #1122, 1000.000000000000000 ) ;
#4961=ORIENTED_EDGE ( 'NONE', *, *, #1945, .T. ) ;
#4962=AXIS2_PLACEMENT_3D ( 'NONE', #277, #1836, #4800 ) ;
ENDSEC;
END-ISO-10303-21;
